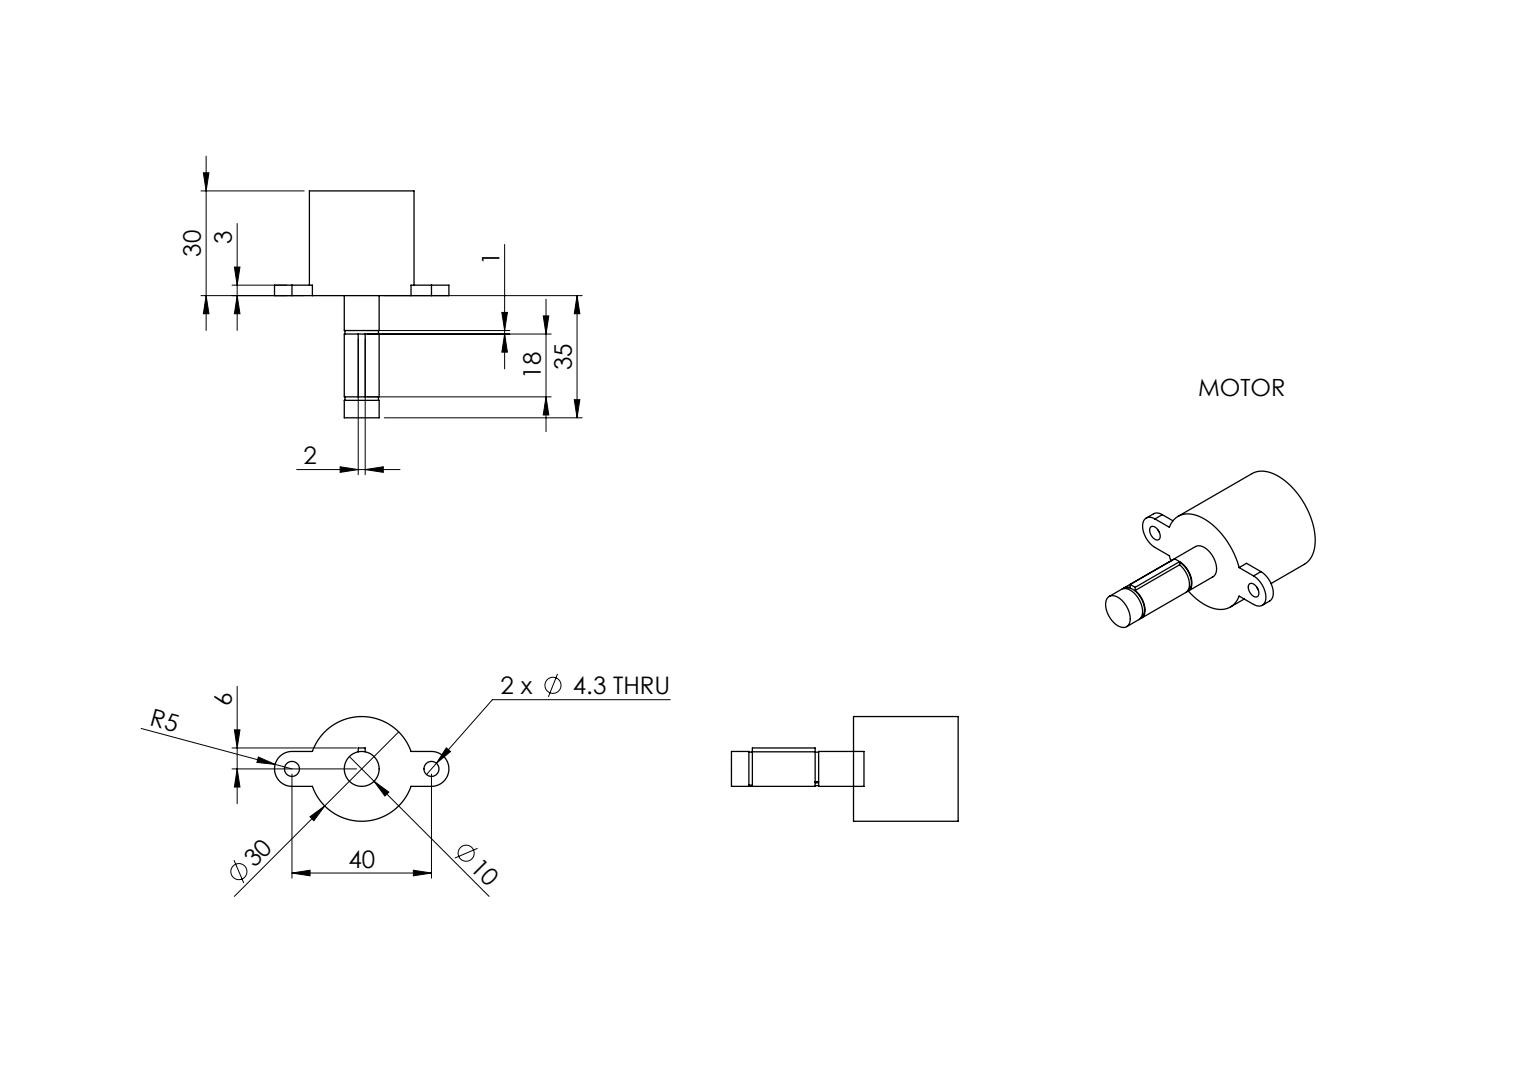
ISO-10303-21;
HEADER;
FILE_DESCRIPTION (('STEP AP214'),
    '1' );
FILE_NAME ('motor.step',
    '2026-10-25T07:12:54',
    ( '' ),
    ( '' ),
    'SwSTEP 2.0',
    'SolidWorks 2026',
    '' );
FILE_SCHEMA (( 'AUTOMOTIVE_DESIGN' ));
ENDSEC;

DATA;
#9=STYLED_ITEM ( 'NONE', ( #1512 ), #12751 ) ;
#21=AXIS2_PLACEMENT_3D ( 'NONE', #13643, #10746, #12742 ) ;
#28=FACE_OUTER_BOUND ( 'NONE', #7057, .T. ) ;
#30=CARTESIAN_POINT ( 'NONE',  ( 22.14999999999999858, -20.00000000000000000, -23.00000000000000000 ) ) ;
#31=ORIENTED_EDGE ( 'NONE', *, *, #5701, .T. ) ;
#100=AXIS2_PLACEMENT_3D ( 'NONE', #7790, #12001, #438 ) ;
#103=EDGE_CURVE ( 'NONE', #12840, #3906, #7426, .T. ) ;
#104=DIRECTION ( 'NONE',  ( -9.710251638871371392E-17, -5.969973981896233748E-17, -1.000000000000000000 ) ) ;
#108=AXIS2_PLACEMENT_3D ( 'NONE', #135, #10772, #2266 ) ;
#110=CARTESIAN_POINT ( 'NONE',  ( 2.385244779468109755E-15, -20.00000000000000000, -9.999999999999994671 ) ) ;
#118=ORIENTED_EDGE ( 'NONE', *, *, #4262, .T. ) ;
#131=ORIENTED_EDGE ( 'NONE', *, *, #11542, .F. ) ;
#135=CARTESIAN_POINT ( 'NONE',  ( 1.267864665261691752E-11, -20.00000000000000000, 9.999999999999998224 ) ) ;
#148=ORIENTED_EDGE ( 'NONE', *, *, #10663, .F. ) ;
#150=ORIENTED_EDGE ( 'NONE', *, *, #2542, .F. ) ;
#159=DIRECTION ( 'NONE',  ( -1.000000000000000000, 0.000000000000000000, 0.000000000000000000 ) ) ;
#171=PLANE ( 'NONE',  #421 ) ;
#179=ORIENTED_EDGE ( 'NONE', *, *, #103, .F. ) ;
#181=ORIENTED_EDGE ( 'NONE', *, *, #4567, .T. ) ;
#190=FACE_OUTER_BOUND ( 'NONE', #6460, .T. ) ;
#202=CARTESIAN_POINT ( 'NONE',  ( -14.99999999999999822, -19.99999999999999645, -23.00000000000000000 ) ) ;
#217=DIRECTION ( 'NONE',  ( -0.000000000000000000, -0.000000000000000000, -1.000000000000000000 ) ) ;
#229=( GEOMETRIC_REPRESENTATION_CONTEXT ( 3 ) GLOBAL_UNCERTAINTY_ASSIGNED_CONTEXT ( ( #8327 ) ) GLOBAL_UNIT_ASSIGNED_CONTEXT ( ( #1931, #1865, #3739 ) ) REPRESENTATION_CONTEXT ( 'NONE', 'WORKASPACE' ) );
#232=ORIENTED_EDGE ( 'NONE', *, *, #13179, .F. ) ;
#250=DIRECTION ( 'NONE',  ( -0.7581610723493046322, -0.6520673188974834833, 1.125475972357111981E-16 ) ) ;
#260=EDGE_CURVE ( 'NONE', #13554, #4523, #9345, .T. ) ;
#263=ORIENTED_EDGE ( 'NONE', *, *, #4115, .F. ) ;
#281=EDGE_CURVE ( 'NONE', #5149, #3301, #7761, .T. ) ;
#283=CYLINDRICAL_SURFACE ( 'NONE', #7915, 5.000000000000000888 ) ;
#294=CARTESIAN_POINT ( 'NONE',  ( 20.00000000000000000, -20.00000000000000000, -23.00000000000000000 ) ) ;
#331=VERTEX_POINT ( 'NONE', #13575 ) ;
#333=LINE ( 'NONE', #7675, #5864 ) ;
#346=ORIENTED_EDGE ( 'NONE', *, *, #2293, .T. ) ;
#347=VERTEX_POINT ( 'NONE', #8345 ) ;
#360=EDGE_CURVE ( 'NONE', #407, #11356, #13500, .T. ) ;
#381=CARTESIAN_POINT ( 'NONE',  ( -3.734041964264191549, -23.01611183630746638, -9.999999999999994671 ) ) ;
#385=CARTESIAN_POINT ( 'NONE',  ( 1.267864665261691752E-11, -20.00000000000000000, 9.999999999999998224 ) ) ;
#405=ORIENTED_EDGE ( 'NONE', *, *, #12351, .T. ) ;
#406=EDGE_LOOP ( 'NONE', ( #1718, #12566, #1882, #5438, #12135, #10903, #5270, #9079, #3095, #9271, #9064, #5318 ) ) ;
#407=VERTEX_POINT ( 'NONE', #11378 ) ;
#421=AXIS2_PLACEMENT_3D ( 'NONE', #8685, #3491, #5379 ) ;
#424=DIRECTION ( 'NONE',  ( 0.6040472319084893016, -0.7969485188038759604, -1.107688701425240097E-17 ) ) ;
#430=AXIS2_PLACEMENT_3D ( 'NONE', #5828, #10990, #3471 ) ;
#435=DIRECTION ( 'NONE',  ( 0.9829867750086872524, 0.1836763462126260182, -1.475957441759982183E-22 ) ) ;
#438=DIRECTION ( 'NONE',  ( -1.000000000000000000, 1.734723475976806848E-16, 0.000000000000000000 ) ) ;
#445=DIRECTION ( 'NONE',  ( 0.000000000000000000, 0.000000000000000000, -1.000000000000000000 ) ) ;
#470=VECTOR ( 'NONE', #11867, 1000.000000000000000 ) ;
#495=CIRCLE ( 'NONE', #6054, 15.00000000000000000 ) ;
#498=DIRECTION ( 'NONE',  ( 1.000000000000000000, 0.000000000000000000, 0.000000000000000000 ) ) ;
#503=EDGE_CURVE ( 'NONE', #347, #12172, #6338, .T. ) ;
#504=VERTEX_POINT ( 'NONE', #30 ) ;
#512=DIRECTION ( 'NONE',  ( -0.000000000000000000, -0.000000000000000000, 1.000000000000000000 ) ) ;
#520=ORIENTED_EDGE ( 'NONE', *, *, #4096, .T. ) ;
#524=CARTESIAN_POINT ( 'NONE',  ( 1.219878473194463187, -24.84890673354692936, 9.000000000000000000 ) ) ;
#538=ORIENTED_EDGE ( 'NONE', *, *, #13172, .T. ) ;
#542=CARTESIAN_POINT ( 'NONE',  ( 20.00000000000000000, -20.00000000000000000, -23.00000000000000000 ) ) ;
#555=CIRCLE ( 'NONE', #9633, 5.000000000000000888 ) ;
#573=DIRECTION ( 'NONE',  ( -0.000000000000000000, -0.000000000000000000, -1.000000000000000000 ) ) ;
#576=LINE ( 'NONE', #13235, #12689 ) ;
#600=DIRECTION ( 'NONE',  ( -0.000000000000000000, -0.000000000000000000, 1.000000000000000000 ) ) ;
#610=CARTESIAN_POINT ( 'NONE',  ( 2.482347295856823136E-15, -20.00000000000000000, -8.999999999999996447 ) ) ;
#623=EDGE_CURVE ( 'NONE', #12722, #6800, #4521, .T. ) ;
#651=VERTEX_POINT ( 'NONE', #1248 ) ;
#653=ORIENTED_EDGE ( 'NONE', *, *, #7184, .F. ) ;
#664=ADVANCED_FACE ( 'NONE', ( #7703 ), #11843, .F. ) ;
#666=VECTOR ( 'NONE', #1055, 1000.000000000000000 ) ;
#683=VECTOR ( 'NONE', #512, 1000.000000000000000 ) ;
#690=VERTEX_POINT ( 'NONE', #9775 ) ;
#692=CIRCLE ( 'NONE', #11545, 2.149999999999999023 ) ;
#705=ORIENTED_EDGE ( 'NONE', *, *, #6210, .F. ) ;
#706=EDGE_CURVE ( 'NONE', #10906, #10425, #3298, .T. ) ;
#711=DIRECTION ( 'NONE',  ( -0.7779254092217071648, -0.6283566325640553840, 0.000000000000000000 ) ) ;
#713=CARTESIAN_POINT ( 'NONE',  ( -4.999999999999998224, -20.00000000000000000, -20.00000000000000000 ) ) ;
#714=DIRECTION ( 'NONE',  ( -0.7779254092217071648, -0.6283566325640553840, 0.000000000000000000 ) ) ;
#728=LINE ( 'NONE', #11257, #8503 ) ;
#735=DIRECTION ( 'NONE',  ( -1.000000000000000000, 0.000000000000000000, 0.000000000000000000 ) ) ;
#739=CIRCLE ( 'NONE', #6941, 5.000000000000000888 ) ;
#742=VECTOR ( 'NONE', #13525, 1000.000000000000000 ) ;
#743=LINE ( 'NONE', #9777, #4835 ) ;
#757=VERTEX_POINT ( 'NONE', #9640 ) ;
#781=CARTESIAN_POINT ( 'NONE',  ( 2.449293598294706513E-15, -20.00000000000000000, -20.00000000000000000 ) ) ;
#784=CARTESIAN_POINT ( 'NONE',  ( 0.8816464618332836567, -24.71833652004169934, 9.999999999999998224 ) ) ;
#790=DIRECTION ( 'NONE',  ( -1.000000000000000000, 0.000000000000000000, 0.000000000000000000 ) ) ;
#800=CARTESIAN_POINT ( 'NONE',  ( 4.688877333453708829, -18.97314589549297281, 9.999999999999998224 ) ) ;
#809=ORIENTED_EDGE ( 'NONE', *, *, #4115, .T. ) ;
#813=CYLINDRICAL_SURFACE ( 'NONE', #10822, 2.149999999999999023 ) ;
#823=ORIENTED_EDGE ( 'NONE', *, *, #3310, .T. ) ;
#824=ORIENTED_EDGE ( 'NONE', *, *, #3992, .T. ) ;
#842=CARTESIAN_POINT ( 'NONE',  ( 14.14213562373095101, -25.00000000000000711, -50.00000000000000000 ) ) ;
#845=ORIENTED_EDGE ( 'NONE', *, *, #3310, .F. ) ;
#849=EDGE_CURVE ( 'NONE', #12479, #12223, #1301, .T. ) ;
#864=EDGE_LOOP ( 'NONE', ( #11730, #7424, #1233, #7744 ) ) ;
#869=CARTESIAN_POINT ( 'NONE',  ( 0.9183817310753817909, -24.91493387504115020, 9.999999999999998224 ) ) ;
#902=DIRECTION ( 'NONE',  ( -1.000000000000000000, 0.000000000000000000, 0.000000000000000000 ) ) ;
#910=EDGE_CURVE ( 'NONE', #11255, #13173, #3889, .T. ) ;
#963=VECTOR ( 'NONE', #11375, 1000.000000000000000 ) ;
#990=ADVANCED_FACE ( 'NONE', ( #9245 ), #7176, .T. ) ;
#995=EDGE_CURVE ( 'NONE', #3770, #10955, #495, .T. ) ;
#1005=DIRECTION ( 'NONE',  ( 0.000000000000000000, 0.000000000000000000, -1.000000000000000000 ) ) ;
#1007=CARTESIAN_POINT ( 'NONE',  ( -20.00000000000000000, -19.99999999999999289, -23.00000000000000000 ) ) ;
#1011=PRODUCT ( 'motor', 'motor', '', ( #7156 ) ) ;
#1012=DIRECTION ( 'NONE',  ( -9.858538378746663627E-23, 5.031452844637890958E-23, -1.000000000000000000 ) ) ;
#1020=CARTESIAN_POINT ( 'NONE',  ( 3.020236159542449172, -23.98474259401938014, -8.999999999999998224 ) ) ;
#1032=EDGE_LOOP ( 'NONE', ( #8046, #6869, #12318, #1285 ) ) ;
#1047=FACE_OUTER_BOUND ( 'NONE', #2834, .T. ) ;
#1048=ORIENTED_EDGE ( 'NONE', *, *, #6072, .F. ) ;
#1055=DIRECTION ( 'NONE',  ( 0.000000000000000000, 0.000000000000000000, 1.000000000000000000 ) ) ;
#1081=ORIENTED_EDGE ( 'NONE', *, *, #7273, .T. ) ;
#1082=ORIENTED_EDGE ( 'NONE', *, *, #503, .T. ) ;
#1084=CARTESIAN_POINT ( 'NONE',  ( 20.00000000000000000, -14.99999999999999289, -20.00000000000000000 ) ) ;
#1088=AXIS2_PLACEMENT_3D ( 'NONE', #1977, #9515, #7322 ) ;
#1102=DIRECTION ( 'NONE',  ( -9.858538378746663627E-23, 5.031452844637890958E-23, -1.000000000000000000 ) ) ;
#1106=DIRECTION ( 'NONE',  ( -1.000000000000000000, 0.000000000000000000, 0.000000000000000000 ) ) ;
#1110=VECTOR ( 'NONE', #8764, 1000.000000000000000 ) ;
#1115=DIRECTION ( 'NONE',  ( 0.000000000000000000, 1.000000000000000000, 0.000000000000000000 ) ) ;
#1139=ORIENTED_EDGE ( 'NONE', *, *, #8132, .T. ) ;
#1170=ORIENTED_EDGE ( 'NONE', *, *, #7701, .F. ) ;
#1175=VECTOR ( 'NONE', #104, 1000.000000000000000 ) ;
#1182=CARTESIAN_POINT ( 'NONE',  ( -17.85000000000000142, -19.99999999999999289, -20.00000000000000000 ) ) ;
#1190=EDGE_LOOP ( 'NONE', ( #2623, #5170, #4957, #13127 ) ) ;
#1199=AXIS2_PLACEMENT_3D ( 'NONE', #9457, #9400, #13594 ) ;
#1203=CARTESIAN_POINT ( 'NONE',  ( 20.00000000000000000, -25.00000000000000711, -23.00000000000000000 ) ) ;
#1204=DIRECTION ( 'NONE',  ( -0.000000000000000000, -0.000000000000000000, -1.000000000000000000 ) ) ;
#1209=EDGE_LOOP ( 'NONE', ( #4886, #9308, #8557, #1048 ) ) ;
#1233=ORIENTED_EDGE ( 'NONE', *, *, #3769, .T. ) ;
#1248=CARTESIAN_POINT ( 'NONE',  ( 1.219878473194463187, -24.84890673354692936, 9.999999999999998224 ) ) ;
#1251=DIRECTION ( 'NONE',  ( -0.2439756946365075896, 0.9697813467099856144, 1.610118993450814692E-22 ) ) ;
#1264=EDGE_LOOP ( 'NONE', ( #3888, #6058, #2553, #520 ) ) ;
#1285=ORIENTED_EDGE ( 'NONE', *, *, #3067, .F. ) ;
#1293=CARTESIAN_POINT ( 'NONE',  ( 5.000000000000003553, -20.00000000000000000, -20.00000000000000000 ) ) ;
#1301=CIRCLE ( 'NONE', #13223, 5.000000000000007994 ) ;
#1306=CARTESIAN_POINT ( 'NONE',  ( 1.267864665261691752E-11, -20.00000000000000000, 9.999999999999998224 ) ) ;
#1322=DIRECTION ( 'NONE',  ( 0.000000000000000000, 0.000000000000000000, -1.000000000000000000 ) ) ;
#1324=CARTESIAN_POINT ( 'NONE',  ( -17.85000000000000142, -19.99999999999999289, -23.00000000000000000 ) ) ;
#1334=ORIENTED_EDGE ( 'NONE', *, *, #4336, .T. ) ;
#1357=CIRCLE ( 'NONE', #4686, 2.149999999999999023 ) ;
#1360=DIRECTION ( 'NONE',  ( -0.7779254092217071648, -0.6283566325640553840, 0.000000000000000000 ) ) ;
#1385=DIRECTION ( 'NONE',  ( 1.000000000000000000, -1.734723475976807341E-16, -0.000000000000000000 ) ) ;
#1388=CARTESIAN_POINT ( 'NONE',  ( 2.899426713160750069, -23.82535289025860337, -9.999999999999994671 ) ) ;
#1395=PLANE ( 'NONE',  #11068 ) ;
#1408=AXIS2_PLACEMENT_3D ( 'NONE', #6301, #1005, #7116 ) ;
#1416=DIRECTION ( 'NONE',  ( 0.6040472319084893016, -0.7969485188038759604, -1.107688701425240251E-17 ) ) ;
#1421=VERTEX_POINT ( 'NONE', #12715 ) ;
#1434=ORIENTED_EDGE ( 'NONE', *, *, #9580, .T. ) ;
#1467=PLANE ( 'NONE',  #5074 ) ;
#1473=ORIENTED_EDGE ( 'NONE', *, *, #11540, .F. ) ;
#1489=VERTEX_POINT ( 'NONE', #2987 ) ;
#1492=FACE_OUTER_BOUND ( 'NONE', #8858, .T. ) ;
#1499=LINE ( 'NONE', #13053, #9995 ) ;
#1512=PRESENTATION_STYLE_ASSIGNMENT (( #6791 ) ) ;
#1546=CARTESIAN_POINT ( 'NONE',  ( -3.734041964264191549, -23.01611183630746638, -8.999999999999996447 ) ) ;
#1555=VECTOR ( 'NONE', #6821, 999.9999999999998863 ) ;
#1574=EDGE_LOOP ( 'NONE', ( #3279, #705, #2695, #5481, #5837, #7241, #9903, #9024 ) ) ;
#1611=EDGE_CURVE ( 'NONE', #13245, #504, #728, .T. ) ;
#1620=AXIS2_PLACEMENT_3D ( 'NONE', #4593, #5570, #8747 ) ;
#1628=AXIS2_PLACEMENT_3D ( 'NONE', #13208, #1322, #6741 ) ;
#1646=ORIENTED_EDGE ( 'NONE', *, *, #12351, .F. ) ;
#1669=CIRCLE ( 'NONE', #5891, 4.799999999999999822 ) ;
#1678=CARTESIAN_POINT ( 'NONE',  ( 20.00000000000000000, -25.00000000000000711, -23.00000000000000000 ) ) ;
#1681=ORIENTED_EDGE ( 'NONE', *, *, #5603, .T. ) ;
#1693=EDGE_CURVE ( 'NONE', #4523, #12971, #6022, .T. ) ;
#1697=EDGE_CURVE ( 'NONE', #5890, #11555, #12498, .T. ) ;
#1704=CARTESIAN_POINT ( 'NONE',  ( 17.85000000000000142, -20.00000000000000000, -23.00000000000000000 ) ) ;
#1708=EDGE_CURVE ( 'NONE', #9272, #8675, #5122, .T. ) ;
#1716=EDGE_LOOP ( 'NONE', ( #232, #7425, #4993, #9885, #7605, #12254, #2606, #5059 ) ) ;
#1718=ORIENTED_EDGE ( 'NONE', *, *, #1708, .F. ) ;
#1719=DIRECTION ( 'NONE',  ( -1.000000000000000000, 0.000000000000000000, 0.000000000000000000 ) ) ;
#1720=LINE ( 'NONE', #9068, #8575 ) ;
#1728=ADVANCED_FACE ( 'NONE', ( #12363 ), #6303, .T. ) ;
#1730=DIRECTION ( 'NONE',  ( -0.2439756946365075896, 0.9697813467099857254, 1.610118993450814692E-22 ) ) ;
#1738=EDGE_LOOP ( 'NONE', ( #9969, #12992 ) ) ;
#1741=SHAPE_DEFINITION_REPRESENTATION ( #12618, #11036 ) ;
#1745=CARTESIAN_POINT ( 'NONE',  ( 2.482347295856823136E-15, -20.00000000000000000, -8.999999999999996447 ) ) ;
#1787=VERTEX_POINT ( 'NONE', #3373 ) ;
#1790=AXIS2_PLACEMENT_3D ( 'NONE', #10437, #10100, #13603 ) ;
#1808=EDGE_LOOP ( 'NONE', ( #1646, #10556, #3839, #4401 ) ) ;
#1819=LINE ( 'NONE', #10329, #2792 ) ;
#1825=AXIS2_PLACEMENT_3D ( 'NONE', #8022, #3667, #7954 ) ;
#1827=EDGE_LOOP ( 'NONE', ( #3789, #7685, #4973, #11985 ) ) ;
#1828=DIRECTION ( 'NONE',  ( 0.000000000000000000, 0.000000000000000000, 1.000000000000000000 ) ) ;
#1840=ORIENTED_EDGE ( 'NONE', *, *, #2185, .F. ) ;
#1844=DIRECTION ( 'NONE',  ( -0.000000000000000000, -0.000000000000000000, -1.000000000000000000 ) ) ;
#1855=CIRCLE ( 'NONE', #5189, 4.800000000000000711 ) ;
#1865=( NAMED_UNIT ( * ) PLANE_ANGLE_UNIT ( ) SI_UNIT ( $, .RADIAN. ) );
#1868=FACE_OUTER_BOUND ( 'NONE', #1808, .T. ) ;
#1880=VECTOR ( 'NONE', #6757, 1000.000000000000000 ) ;
#1882=ORIENTED_EDGE ( 'NONE', *, *, #8132, .F. ) ;
#1885=CARTESIAN_POINT ( 'NONE',  ( 2.449293598294706513E-15, -20.00000000000000000, 15.00000000000000355 ) ) ;
#1896=DIRECTION ( 'NONE',  ( -1.000000000000000000, 0.000000000000000000, 0.000000000000000000 ) ) ;
#1897=ORIENTED_EDGE ( 'NONE', *, *, #7519, .T. ) ;
#1899=DIRECTION ( 'NONE',  ( 1.000000000000000000, 0.000000000000000000, 0.000000000000000000 ) ) ;
#1916=DIRECTION ( 'NONE',  ( -1.000000000000000000, 0.000000000000000000, 0.000000000000000000 ) ) ;
#1930=VECTOR ( 'NONE', #7556, 1000.000000000000000 ) ;
#1931=( LENGTH_UNIT ( ) NAMED_UNIT ( * ) SI_UNIT ( .MILLI., .METRE. ) );
#1937=ADVANCED_FACE ( 'NONE', ( #6562, #10762, #4278, #11609 ), #6367, .F. ) ;
#1941=ORIENTED_EDGE ( 'NONE', *, *, #3233, .F. ) ;
#1950=DIRECTION ( 'NONE',  ( 0.000000000000000000, 0.000000000000000000, -1.000000000000000000 ) ) ;
#1972=AXIS2_PLACEMENT_3D ( 'NONE', #3079, #6284, #1896 ) ;
#1977=CARTESIAN_POINT ( 'NONE',  ( 2.449293598294706513E-15, -20.00000000000000000, 15.00000000000000355 ) ) ;
#1987=FACE_OUTER_BOUND ( 'NONE', #1190, .T. ) ;
#1988=AXIS2_PLACEMENT_3D ( 'NONE', #7337, #1012, #3309 ) ;
#1989=ORIENTED_EDGE ( 'NONE', *, *, #11540, .T. ) ;
#2013=EDGE_CURVE ( 'NONE', #5545, #4887, #2463, .T. ) ;
#2015=ORIENTED_EDGE ( 'NONE', *, *, #2346, .F. ) ;
#2034=CYLINDRICAL_SURFACE ( 'NONE', #5843, 4.800000000000000711 ) ;
#2042=CYLINDRICAL_SURFACE ( 'NONE', #21, 4.799999999999999822 ) ;
#2070=CARTESIAN_POINT ( 'NONE',  ( -0.9999999999999995559, -15.10102051443364246, 15.00000000000000355 ) ) ;
#2088=AXIS2_PLACEMENT_3D ( 'NONE', #10550, #3091, #790 ) ;
#2098=CARTESIAN_POINT ( 'NONE',  ( 1.267864665261691752E-11, -20.00000000000000000, 9.999999999999998224 ) ) ;
#2109=EDGE_CURVE ( 'NONE', #10425, #12479, #6894, .T. ) ;
#2134=CARTESIAN_POINT ( 'NONE',  ( 2.899426713160750069, -23.82535289025860337, -8.999999999999996447 ) ) ;
#2169=FACE_OUTER_BOUND ( 'NONE', #7043, .T. ) ;
#2181=EDGE_LOOP ( 'NONE', ( #3330, #12040, #2890, #2015 ) ) ;
#2185=EDGE_CURVE ( 'NONE', #1787, #12223, #12747, .T. ) ;
#2188=FACE_OUTER_BOUND ( 'NONE', #13311, .T. ) ;
#2214=AXIS2_PLACEMENT_3D ( 'NONE', #10842, #9748, #7676 ) ;
#2225=CARTESIAN_POINT ( 'NONE',  ( 17.85000000000000142, -20.00000000000000000, -23.00000000000000000 ) ) ;
#2233=CARTESIAN_POINT ( 'NONE',  ( 14.14213562373095101, -25.00000000000000711, -23.00000000000000000 ) ) ;
#2234=AXIS2_PLACEMENT_3D ( 'NONE', #7626, #8735, #6727 ) ;
#2242=DIRECTION ( 'NONE',  ( -1.000000000000000000, 0.000000000000000000, 0.000000000000000000 ) ) ;
#2266=DIRECTION ( 'NONE',  ( -0.9768494444668812671, -0.2139279384389642935, 0.000000000000000000 ) ) ;
#2267=CARTESIAN_POINT ( 'NONE',  ( -1.000000000000000000, -14.00000000000000000, 8.999999999999998224 ) ) ;
#2282=ADVANCED_FACE ( 'NONE', ( #10880 ), #1395, .F. ) ;
#2284=CIRCLE ( 'NONE', #10239, 5.000000000000007994 ) ;
#2290=EDGE_CURVE ( 'NONE', #6976, #8572, #4455, .T. ) ;
#2293=EDGE_CURVE ( 'NONE', #11760, #5079, #4909, .T. ) ;
#2298=VECTOR ( 'NONE', #9222, 1000.000000000000000 ) ;
#2300=ADVANCED_FACE ( 'NONE', ( #11997 ), #12882, .T. ) ;
#2305=DIRECTION ( 'NONE',  ( -0.9697813467099857254, -0.2439756946365076173, 1.379242460255691792E-22 ) ) ;
#2346=EDGE_CURVE ( 'NONE', #4780, #6905, #13357, .T. ) ;
#2347=ORIENTED_EDGE ( 'NONE', *, *, #10264, .F. ) ;
#2349=ORIENTED_EDGE ( 'NONE', *, *, #7292, .F. ) ;
#2392=AXIS2_PLACEMENT_3D ( 'NONE', #10166, #11198, #1719 ) ;
#2400=ORIENTED_EDGE ( 'NONE', *, *, #13346, .F. ) ;
#2420=VECTOR ( 'NONE', #2954, 1000.000000000000000 ) ;
#2427=EDGE_CURVE ( 'NONE', #5888, #11823, #1669, .T. ) ;
#2432=AXIS2_PLACEMENT_3D ( 'NONE', #6382, #10446, #3255 ) ;
#2437=DIRECTION ( 'NONE',  ( -0.000000000000000000, -0.000000000000000000, -1.000000000000000000 ) ) ;
#2463=CIRCLE ( 'NONE', #3137, 2.149999999999999023 ) ;
#2500=DIRECTION ( 'NONE',  ( -1.734723475976807341E-16, -1.000000000000000000, 0.000000000000000000 ) ) ;
#2521=AXIS2_PLACEMENT_3D ( 'NONE', #1007, #9459, #8431 ) ;
#2526=CARTESIAN_POINT ( 'NONE',  ( 5.000000000000003553, -20.00000000000000000, -9.999999999999994671 ) ) ;
#2529=EDGE_CURVE ( 'NONE', #4887, #5545, #12500, .T. ) ;
#2542=EDGE_CURVE ( 'NONE', #9150, #5892, #555, .T. ) ;
#2543=DIRECTION ( 'NONE',  ( 0.000000000000000000, 0.000000000000000000, -1.000000000000000000 ) ) ;
#2553=ORIENTED_EDGE ( 'NONE', *, *, #10454, .T. ) ;
#2556=ORIENTED_EDGE ( 'NONE', *, *, #4759, .F. ) ;
#2562=SURFACE_SIDE_STYLE ('',( #8865 ) ) ;
#2569=CARTESIAN_POINT ( 'NONE',  ( 20.00000000000000000, -14.99999999999999289, -23.00000000000000000 ) ) ;
#2574=CARTESIAN_POINT ( 'NONE',  ( 20.00000000000000000, -20.00000000000000000, -20.00000000000000000 ) ) ;
#2578=CARTESIAN_POINT ( 'NONE',  ( 1.267864665251833278E-11, -20.00000000000000000, 9.000000000000000000 ) ) ;
#2583=DIRECTION ( 'NONE',  ( -0.7779254092217071648, -0.6283566325640553840, 0.000000000000000000 ) ) ;
#2591=DIRECTION ( 'NONE',  ( -1.000000000000000000, 0.000000000000000000, 0.000000000000000000 ) ) ;
#2603=AXIS2_PLACEMENT_3D ( 'NONE', #8934, #600, #13263 ) ;
#2606=ORIENTED_EDGE ( 'NONE', *, *, #995, .T. ) ;
#2614=CYLINDRICAL_SURFACE ( 'NONE', #6233, 15.00000000000000000 ) ;
#2622=AXIS2_PLACEMENT_3D ( 'NONE', #11016, #12266, #3968 ) ;
#2623=ORIENTED_EDGE ( 'NONE', *, *, #1697, .T. ) ;
#2624=ORIENTED_EDGE ( 'NONE', *, *, #6395, .T. ) ;
#2659=ORIENTED_EDGE ( 'NONE', *, *, #2719, .T. ) ;
#2677=VERTEX_POINT ( 'NONE', #13569 ) ;
#2680=ORIENTED_EDGE ( 'NONE', *, *, #4096, .F. ) ;
#2695=ORIENTED_EDGE ( 'NONE', *, *, #7552, .T. ) ;
#2697=ORIENTED_EDGE ( 'NONE', *, *, #8399, .T. ) ;
#2698=DIRECTION ( 'NONE',  ( -0.000000000000000000, -0.000000000000000000, 1.000000000000000000 ) ) ;
#2711=VERTEX_POINT ( 'NONE', #9229 ) ;
#2719=EDGE_CURVE ( 'NONE', #11823, #11760, #1819, .T. ) ;
#2746=AXIS2_PLACEMENT_3D ( 'NONE', #11584, #1115, #13429 ) ;
#2755=ORIENTED_EDGE ( 'NONE', *, *, #12525, .T. ) ;
#2771=VERTEX_POINT ( 'NONE', #1182 ) ;
#2789=VERTEX_POINT ( 'NONE', #5559 ) ;
#2792=VECTOR ( 'NONE', #6065, 1000.000000000000114 ) ;
#2813=CARTESIAN_POINT ( 'NONE',  ( 2.449293598294706513E-15, -20.00000000000000000, -23.00000000000000000 ) ) ;
#2834=EDGE_LOOP ( 'NONE', ( #10782, #13044, #1897, #7724 ) ) ;
#2840=FACE_OUTER_BOUND ( 'NONE', #9132, .T. ) ;
#2850=AXIS2_PLACEMENT_3D ( 'NONE', #8753, #11789, #9651 ) ;
#2853=DIRECTION ( 'NONE',  ( 0.000000000000000000, 0.000000000000000000, -1.000000000000000000 ) ) ;
#2870=DIRECTION ( 'NONE',  ( -0.000000000000000000, -0.000000000000000000, 1.000000000000000000 ) ) ;
#2890=ORIENTED_EDGE ( 'NONE', *, *, #10531, .T. ) ;
#2891=CARTESIAN_POINT ( 'NONE',  ( 20.00000000000000000, -14.99999999999999289, -23.00000000000000000 ) ) ;
#2900=DIRECTION ( 'NONE',  ( -0.000000000000000000, -0.000000000000000000, 1.000000000000000000 ) ) ;
#2908=ORIENTED_EDGE ( 'NONE', *, *, #3602, .T. ) ;
#2912=FACE_BOUND ( 'NONE', #1738, .T. ) ;
#2936=CARTESIAN_POINT ( 'NONE',  ( -22.14999999999999858, -19.99999999999999289, -23.00000000000000000 ) ) ;
#2943=CIRCLE ( 'NONE', #1825, 5.000000000000000888 ) ;
#2949=DIRECTION ( 'NONE',  ( -1.000000000000000000, -4.082155997157843695E-16, 0.000000000000000000 ) ) ;
#2950=CLOSED_SHELL ( 'NONE', ( #6174, #8344, #9664, #6098, #2981, #7491, #8600, #10497, #7205, #10910, #2300, #9930, #10273, #9322, #11759, #1937, #1728, #8370, #10770, #3896, #7071, #10494, #5349, #10066, #7769, #664, #7458, #4338, #6200, #6808, #7135, #9712, #2282, #990, #13011, #6166, #10063, #4236, #5363, #5115 ) ) ;
#2954=DIRECTION ( 'NONE',  ( -9.858538378746663627E-23, 5.031452844637890958E-23, -1.000000000000000000 ) ) ;
#2974=VECTOR ( 'NONE', #8259, 1000.000000000000000 ) ;
#2981=ADVANCED_FACE ( 'NONE', ( #4725 ), #5835, .T. ) ;
#2987=CARTESIAN_POINT ( 'NONE',  ( -20.00000000000000000, -25.00000000000000000, -20.00000000000000000 ) ) ;
#3018=PLANE ( 'NONE',  #6000 ) ;
#3026=ORIENTED_EDGE ( 'NONE', *, *, #9719, .T. ) ;
#3031=CARTESIAN_POINT ( 'NONE',  ( 2.449293598294706513E-15, -20.00000000000000000, -20.00000000000000000 ) ) ;
#3054=VECTOR ( 'NONE', #7812, 1000.000000000000000 ) ;
#3062=CARTESIAN_POINT ( 'NONE',  ( -4.999999999999998224, -20.00000000000000000, 15.00000000000000355 ) ) ;
#3067=EDGE_CURVE ( 'NONE', #690, #1489, #13074, .T. ) ;
#3077=ORIENTED_EDGE ( 'NONE', *, *, #13406, .T. ) ;
#3079=CARTESIAN_POINT ( 'NONE',  ( 2.449293598294706513E-15, -20.00000000000000000, 9.000000000000000000 ) ) ;
#3082=ORIENTED_EDGE ( 'NONE', *, *, #5188, .F. ) ;
#3083=CARTESIAN_POINT ( 'NONE',  ( 2.449293598294706513E-15, -20.00000000000000000, -23.00000000000000000 ) ) ;
#3085=DIRECTION ( 'NONE',  ( -9.858538378746663627E-23, 5.031452844637890958E-23, -1.000000000000000000 ) ) ;
#3091=DIRECTION ( 'NONE',  ( -9.710251638871371392E-17, -5.969973981896233748E-17, -1.000000000000000000 ) ) ;
#3095=ORIENTED_EDGE ( 'NONE', *, *, #503, .F. ) ;
#3137=AXIS2_PLACEMENT_3D ( 'NONE', #6761, #573, #9994 ) ;
#3147=VERTEX_POINT ( 'NONE', #10178 ) ;
#3170=EDGE_CURVE ( 'NONE', #10837, #331, #11981, .T. ) ;
#3179=AXIS2_PLACEMENT_3D ( 'NONE', #11237, #4962, #711 ) ;
#3218=ORIENTED_EDGE ( 'NONE', *, *, #13008, .F. ) ;
#3233=EDGE_CURVE ( 'NONE', #7327, #9150, #8320, .T. ) ;
#3234=ORIENTED_EDGE ( 'NONE', *, *, #623, .F. ) ;
#3239=CARTESIAN_POINT ( 'NONE',  ( 1.171083334267915221, -24.65495046420793201, 9.000000000000000000 ) ) ;
#3246=EDGE_CURVE ( 'NONE', #331, #10837, #4038, .T. ) ;
#3255=DIRECTION ( 'NONE',  ( -1.000000000000000000, 0.000000000000000000, 0.000000000000000000 ) ) ;
#3265=EDGE_LOOP ( 'NONE', ( #8290, #11231, #5908, #5824 ) ) ;
#3279=ORIENTED_EDGE ( 'NONE', *, *, #11433, .F. ) ;
#3280=CARTESIAN_POINT ( 'NONE',  ( 1.000000000000002442, -20.00000000000000000, 8.999999999999998224 ) ) ;
#3291=DIRECTION ( 'NONE',  ( -9.710251638871371392E-17, -5.969973981896234981E-17, -1.000000000000000000 ) ) ;
#3298=CIRCLE ( 'NONE', #12126, 5.000000000000007994 ) ;
#3300=VERTEX_POINT ( 'NONE', #7481 ) ;
#3301=VERTEX_POINT ( 'NONE', #8449 ) ;
#3309=DIRECTION ( 'NONE',  ( -1.000000000000000000, 0.000000000000000000, 0.000000000000000000 ) ) ;
#3310=EDGE_CURVE ( 'NONE', #757, #1421, #12783, .T. ) ;
#3330=ORIENTED_EDGE ( 'NONE', *, *, #10658, .F. ) ;
#3331=EDGE_LOOP ( 'NONE', ( #9117, #10285, #6836, #2680, #3234, #8758, #8426, #4013, #8427 ) ) ;
#3342=CARTESIAN_POINT ( 'NONE',  ( 3.734041964264196878, -16.98388816369253362, -8.999999999999996447 ) ) ;
#3352=CARTESIAN_POINT ( 'NONE',  ( 1.171083334267915221, -24.65495046420793201, 9.999999999999998224 ) ) ;
#3353=AXIS2_PLACEMENT_3D ( 'NONE', #10621, #6487, #3428 ) ;
#3373=CARTESIAN_POINT ( 'NONE',  ( 20.00000000000000000, -25.00000000000000711, -23.00000000000000000 ) ) ;
#3380=AXIS2_PLACEMENT_3D ( 'NONE', #1306, #6461, #10724 ) ;
#3386=DIRECTION ( 'NONE',  ( -0.000000000000000000, -0.000000000000000000, -1.000000000000000000 ) ) ;
#3408=CIRCLE ( 'NONE', #7837, 5.000000000000007994 ) ;
#3428=DIRECTION ( 'NONE',  ( -1.000000000000000000, 0.000000000000000000, 0.000000000000000000 ) ) ;
#3431=DIRECTION ( 'NONE',  ( -1.000000000000000000, 0.000000000000000000, 0.000000000000000000 ) ) ;
#3458=CARTESIAN_POINT ( 'NONE',  ( -1.000000000000000000, -14.00000000000000000, 8.999999999999998224 ) ) ;
#3462=CARTESIAN_POINT ( 'NONE',  ( 3.129923130707922496, -23.63917314727666152, -8.999999999999996447 ) ) ;
#3470=LINE ( 'NONE', #7762, #1930 ) ;
#3471=DIRECTION ( 'NONE',  ( 1.000000000000000000, 0.000000000000000000, 0.000000000000000000 ) ) ;
#3479=EDGE_CURVE ( 'NONE', #10164, #7327, #2943, .T. ) ;
#3491=DIRECTION ( 'NONE',  ( -1.545477659731174253E-22, 3.805888647522192075E-23, -1.000000000000000000 ) ) ;
#3500=ORIENTED_EDGE ( 'NONE', *, *, #13206, .F. ) ;
#3502=CIRCLE ( 'NONE', #11460, 5.000000000000000888 ) ;
#3517=EDGE_LOOP ( 'NONE', ( #5686, #6143 ) ) ;
#3528=CIRCLE ( 'NONE', #9706, 4.799999999999999822 ) ;
#3544=APPLICATION_CONTEXT ( 'automotive_design' ) ;
#3556=VECTOR ( 'NONE', #9975, 1000.000000000000000 ) ;
#3560=EDGE_CURVE ( 'NONE', #9611, #13146, #1499, .T. ) ;
#3588=CARTESIAN_POINT ( 'NONE',  ( 1.000000000000002442, -20.00000000000000000, 8.999999999999998224 ) ) ;
#3602=EDGE_CURVE ( 'NONE', #6107, #9574, #6492, .T. ) ;
#3611=DIRECTION ( 'NONE',  ( 1.000000000000000000, -1.734723475976807341E-16, -0.000000000000000000 ) ) ;
#3615=DIRECTION ( 'NONE',  ( 9.710251638871371392E-17, 5.969973981896233748E-17, 1.000000000000000000 ) ) ;
#3644=CARTESIAN_POINT ( 'NONE',  ( -20.00000000000000000, -19.99999999999999289, -20.00000000000000000 ) ) ;
#3656=EDGE_LOOP ( 'NONE', ( #12645, #6036, #4122, #11341 ) ) ;
#3667=DIRECTION ( 'NONE',  ( -9.710251638871371392E-17, -5.969973981896233748E-17, -1.000000000000000000 ) ) ;
#3688=CARTESIAN_POINT ( 'NONE',  ( -14.14213562373094213, -14.99999999999998757, -23.00000000000000000 ) ) ;
#3702=CARTESIAN_POINT ( 'NONE',  ( 15.00000000000000178, -20.00000000000000000, -23.00000000000000000 ) ) ;
#3705=CARTESIAN_POINT ( 'NONE',  ( 2.449293598294706513E-15, -20.00000000000000000, 15.00000000000000355 ) ) ;
#3718=CARTESIAN_POINT ( 'NONE',  ( -14.14213562373094213, -14.99999999999998757, -50.00000000000000000 ) ) ;
#3739=( NAMED_UNIT ( * ) SI_UNIT ( $, .STERADIAN. ) SOLID_ANGLE_UNIT ( ) );
#3742=EDGE_CURVE ( 'NONE', #12223, #407, #10368, .T. ) ;
#3755=EDGE_LOOP ( 'NONE', ( #3082, #10073, #824, #6572, #8824, #1139, #9357, #10974, #1989, #6075, #5455, #8743, #1941, #5042, #12056, #6328, #5172, #1082, #5616, #9808 ) ) ;
#3757=DIRECTION ( 'NONE',  ( -1.000000000000000000, 0.000000000000000000, 0.000000000000000000 ) ) ;
#3769=EDGE_CURVE ( 'NONE', #1421, #2711, #5056, .T. ) ;
#3770=VERTEX_POINT ( 'NONE', #4081 ) ;
#3781=DIRECTION ( 'NONE',  ( 1.000000000000000000, 0.000000000000000000, 0.000000000000000000 ) ) ;
#3789=ORIENTED_EDGE ( 'NONE', *, *, #6654, .F. ) ;
#3792=VECTOR ( 'NONE', #11808, 999.9999999999998863 ) ;
#3817=EDGE_CURVE ( 'NONE', #2789, #757, #8823, .T. ) ;
#3819=AXIS2_PLACEMENT_3D ( 'NONE', #8180, #5218, #3884 ) ;
#3834=CARTESIAN_POINT ( 'NONE',  ( -20.00000000000000000, -19.99999999999999289, -23.00000000000000000 ) ) ;
#3837=DIRECTION ( 'NONE',  ( 0.000000000000000000, 0.000000000000000000, -1.000000000000000000 ) ) ;
#3839=ORIENTED_EDGE ( 'NONE', *, *, #10737, .T. ) ;
#3844=CARTESIAN_POINT ( 'NONE',  ( -3.734041964264191549, -23.01611183630746638, -8.999999999999996447 ) ) ;
#3860=ORIENTED_EDGE ( 'NONE', *, *, #11926, .T. ) ;
#3884=DIRECTION ( 'NONE',  ( 1.000000000000000000, 0.000000000000000000, 0.000000000000000000 ) ) ;
#3888=ORIENTED_EDGE ( 'NONE', *, *, #2109, .F. ) ;
#3889=LINE ( 'NONE', #7077, #9049 ) ;
#3890=ORIENTED_EDGE ( 'NONE', *, *, #11945, .T. ) ;
#3893=DIRECTION ( 'NONE',  ( 0.000000000000000000, 0.000000000000000000, -1.000000000000000000 ) ) ;
#3896=ADVANCED_FACE ( 'NONE', ( #4605 ), #11925, .F. ) ;
#3901=CYLINDRICAL_SURFACE ( 'NONE', #5733, 2.149999999999999023 ) ;
#3906=VERTEX_POINT ( 'NONE', #12819 ) ;
#3913=( NAMED_UNIT ( * ) PLANE_ANGLE_UNIT ( ) SI_UNIT ( $, .RADIAN. ) );
#3927=DIRECTION ( 'NONE',  ( -1.000000000000000000, 0.000000000000000000, 0.000000000000000000 ) ) ;
#3944=CARTESIAN_POINT ( 'NONE',  ( 2.449293598294706513E-15, -20.00000000000000000, -8.999999999999998224 ) ) ;
#3954=CIRCLE ( 'NONE', #12776, 15.00000000000000000 ) ;
#3956=ORIENTED_EDGE ( 'NONE', *, *, #706, .T. ) ;
#3957=ORIENTED_EDGE ( 'NONE', *, *, #5425, .F. ) ;
#3968=DIRECTION ( 'NONE',  ( -1.000000000000000000, 0.000000000000000000, -0.000000000000000000 ) ) ;
#3980=CARTESIAN_POINT ( 'NONE',  ( -0.9999999999999976685, -20.00000000000000000, 8.999999999999998224 ) ) ;
#3992=EDGE_CURVE ( 'NONE', #10837, #6107, #10267, .T. ) ;
#4009=DIRECTION ( 'NONE',  ( -9.710251638871371392E-17, -5.969973981896233748E-17, -1.000000000000000000 ) ) ;
#4013=ORIENTED_EDGE ( 'NONE', *, *, #7273, .F. ) ;
#4026=AXIS2_PLACEMENT_3D ( 'NONE', #11640, #8598, #159 ) ;
#4038=CIRCLE ( 'NONE', #3819, 5.000000000000000888 ) ;
#4069=ORIENTED_EDGE ( 'NONE', *, *, #1693, .T. ) ;
#4079=LINE ( 'NONE', #4933, #10199 ) ;
#4081=CARTESIAN_POINT ( 'NONE',  ( 14.14213562373094923, -14.99999999999999112, -23.00000000000000000 ) ) ;
#4096=EDGE_CURVE ( 'NONE', #6800, #12479, #3408, .T. ) ;
#4115=EDGE_CURVE ( 'NONE', #1787, #11356, #5856, .T. ) ;
#4119=EDGE_LOOP ( 'NONE', ( #2349, #3077, #4694, #5133 ) ) ;
#4122=ORIENTED_EDGE ( 'NONE', *, *, #2013, .T. ) ;
#4128=DIRECTION ( 'NONE',  ( 4.082155997157843695E-16, -1.000000000000000000, 0.000000000000000000 ) ) ;
#4129=( LENGTH_UNIT ( ) NAMED_UNIT ( * ) SI_UNIT ( .MILLI., .METRE. ) );
#4163=EDGE_CURVE ( 'NONE', #11255, #5890, #13090, .T. ) ;
#4191=CARTESIAN_POINT ( 'NONE',  ( 3.020236159542449172, -23.98474259401938014, -9.999999999999994671 ) ) ;
#4208=PLANE ( 'NONE',  #4663 ) ;
#4214=VECTOR ( 'NONE', #3611, 1000.000000000000000 ) ;
#4219=EDGE_CURVE ( 'NONE', #4643, #12840, #4296, .T. ) ;
#4236=ADVANCED_FACE ( 'NONE', ( #1047 ), #2034, .T. ) ;
#4246=LINE ( 'NONE', #8464, #5347 ) ;
#4260=CARTESIAN_POINT ( 'NONE',  ( 2.899426713160750069, -23.82535289025860337, -8.999999999999996447 ) ) ;
#4262=EDGE_CURVE ( 'NONE', #9574, #651, #739, .T. ) ;
#4277=DIRECTION ( 'NONE',  ( 0.000000000000000000, 0.000000000000000000, -1.000000000000000000 ) ) ;
#4278=FACE_BOUND ( 'NONE', #9027, .T. ) ;
#4285=AXIS2_PLACEMENT_3D ( 'NONE', #3352, #2305, #1251 ) ;
#4286=ORIENTED_EDGE ( 'NONE', *, *, #4219, .T. ) ;
#4296=CIRCLE ( 'NONE', #12677, 4.800000000000000711 ) ;
#4321=ORIENTED_EDGE ( 'NONE', *, *, #3067, .T. ) ;
#4325=LINE ( 'NONE', #10615, #11944 ) ;
#4336=EDGE_CURVE ( 'NONE', #13537, #4887, #6209, .T. ) ;
#4338=ADVANCED_FACE ( 'NONE', ( #28 ), #7375, .T. ) ;
#4353=ORIENTED_EDGE ( 'NONE', *, *, #12603, .T. ) ;
#4385=FACE_OUTER_BOUND ( 'NONE', #6922, .T. ) ;
#4392=CARTESIAN_POINT ( 'NONE',  ( -4.999999999999998224, -20.00000000000000000, 9.999999999999998224 ) ) ;
#4401=ORIENTED_EDGE ( 'NONE', *, *, #5192, .F. ) ;
#4423=CARTESIAN_POINT ( 'NONE',  ( -4.688877333428352223, -21.02685410450703074, 9.000000000000000000 ) ) ;
#4431=ORIENTED_EDGE ( 'NONE', *, *, #7807, .F. ) ;
#4436=DIRECTION ( 'NONE',  ( -1.000000000000000000, 0.000000000000000000, 0.000000000000000000 ) ) ;
#4449=DIRECTION ( 'NONE',  ( 0.000000000000000000, 0.000000000000000000, -1.000000000000000000 ) ) ;
#4450=EDGE_LOOP ( 'NONE', ( #12237, #8510, #6723, #653 ) ) ;
#4454=CARTESIAN_POINT ( 'NONE',  ( 4.688877333453707941, -18.97314589549297281, 9.000000000000000000 ) ) ;
#4455=CIRCLE ( 'NONE', #7548, 4.799999999999999822 ) ;
#4478=AXIS2_PLACEMENT_3D ( 'NONE', #10451, #11281, #8251 ) ;
#4502=EDGE_LOOP ( 'NONE', ( #13380, #7746, #3956, #11568, #809, #6852 ) ) ;
#4512=VECTOR ( 'NONE', #6814, 1000.000000000000000 ) ;
#4515=DIRECTION ( 'NONE',  ( -0.000000000000000000, -0.000000000000000000, -1.000000000000000000 ) ) ;
#4521=LINE ( 'NONE', #10870, #8597 ) ;
#4523=VERTEX_POINT ( 'NONE', #12283 ) ;
#4541=ORIENTED_EDGE ( 'NONE', *, *, #13352, .F. ) ;
#4567=EDGE_CURVE ( 'NONE', #8675, #4780, #7871, .T. ) ;
#4593=CARTESIAN_POINT ( 'NONE',  ( 2.449293598294706513E-15, -20.00000000000000000, -9.999999999999994671 ) ) ;
#4601=CARTESIAN_POINT ( 'NONE',  ( 2.449293598294706513E-15, -20.00000000000000000, -8.999999999999998224 ) ) ;
#4605=FACE_OUTER_BOUND ( 'NONE', #1032, .T. ) ;
#4620=EDGE_CURVE ( 'NONE', #10162, #6905, #576, .T. ) ;
#4621=DIRECTION ( 'NONE',  ( -4.082155997157844188E-16, 1.000000000000000000, 0.000000000000000000 ) ) ;
#4643=VERTEX_POINT ( 'NONE', #8486 ) ;
#4653=CYLINDRICAL_SURFACE ( 'NONE', #13272, 2.149999999999999023 ) ;
#4663=AXIS2_PLACEMENT_3D ( 'NONE', #12635, #250, #10560 ) ;
#4686=AXIS2_PLACEMENT_3D ( 'NONE', #8339, #12471, #13494 ) ;
#4694=ORIENTED_EDGE ( 'NONE', *, *, #623, .T. ) ;
#4714=ORIENTED_EDGE ( 'NONE', *, *, #12713, .T. ) ;
#4717=DIRECTION ( 'NONE',  ( -1.000000000000000000, 1.734723475976806848E-16, 0.000000000000000000 ) ) ;
#4725=FACE_OUTER_BOUND ( 'NONE', #4450, .T. ) ;
#4739=DIRECTION ( 'NONE',  ( -1.000000000000000000, 0.000000000000000000, 0.000000000000000000 ) ) ;
#4750=CARTESIAN_POINT ( 'NONE',  ( 0.8816464618332836567, -24.71833652004169934, 9.999999999999998224 ) ) ;
#4759=EDGE_CURVE ( 'NONE', #7327, #2789, #8724, .T. ) ;
#4780=VERTEX_POINT ( 'NONE', #7248 ) ;
#4784=LINE ( 'NONE', #13134, #4214 ) ;
#4799=DIRECTION ( 'NONE',  ( -0.7779254092217071648, -0.6283566325640553840, 0.000000000000000000 ) ) ;
#4809=DIRECTION ( 'NONE',  ( -1.000000000000000000, 0.000000000000000000, 0.000000000000000000 ) ) ;
#4835=VECTOR ( 'NONE', #2437, 1000.000000000000000 ) ;
#4845=AXIS2_PLACEMENT_3D ( 'NONE', #7274, #11557, #13540 ) ;
#4852=SHAPE_REPRESENTATION_RELATIONSHIP ( 'NONE' , 'NONE' ,  #11036, #12751 ) ;
#4877=MECHANICAL_DESIGN_GEOMETRIC_PRESENTATION_REPRESENTATION('',(#9),#229);
#4886=ORIENTED_EDGE ( 'NONE', *, *, #7173, .F. ) ;
#4887=VERTEX_POINT ( 'NONE', #2936 ) ;
#4906=LINE ( 'NONE', #3718, #12469 ) ;
#4909=CIRCLE ( 'NONE', #10420, 5.000000000000000888 ) ;
#4925=PLANE ( 'NONE',  #9241 ) ;
#4933=CARTESIAN_POINT ( 'NONE',  ( 1.171083334267915221, -24.65495046420793201, 9.000000000000000000 ) ) ;
#4938=ORIENTED_EDGE ( 'NONE', *, *, #12761, .T. ) ;
#4950=DIRECTION ( 'NONE',  ( 9.710251638871371392E-17, 5.969973981896233748E-17, 1.000000000000000000 ) ) ;
#4957=ORIENTED_EDGE ( 'NONE', *, *, #910, .F. ) ;
#4962=DIRECTION ( 'NONE',  ( 9.710251638871371392E-17, 5.969973981896233748E-17, 1.000000000000000000 ) ) ;
#4972=AXIS2_PLACEMENT_3D ( 'NONE', #10561, #5323, #9529 ) ;
#4973=ORIENTED_EDGE ( 'NONE', *, *, #9143, .T. ) ;
#4975=CIRCLE ( 'NONE', #6736, 2.149999999999999023 ) ;
#4979=VERTEX_POINT ( 'NONE', #11435 ) ;
#4991=EDGE_LOOP ( 'NONE', ( #10372, #3860, #3957, #13130 ) ) ;
#4993=ORIENTED_EDGE ( 'NONE', *, *, #13346, .T. ) ;
#4995=CARTESIAN_POINT ( 'NONE',  ( 25.00000000000000711, -20.00000000000000000, -23.00000000000000000 ) ) ;
#5008=ORIENTED_EDGE ( 'NONE', *, *, #2290, .T. ) ;
#5024=PLANE ( 'NONE',  #2622 ) ;
#5042=ORIENTED_EDGE ( 'NONE', *, *, #4759, .T. ) ;
#5050=DIRECTION ( 'NONE',  ( -9.858538378746663627E-23, 5.031452844637890958E-23, -1.000000000000000000 ) ) ;
#5056=LINE ( 'NONE', #13460, #7144 ) ;
#5059=ORIENTED_EDGE ( 'NONE', *, *, #7552, .F. ) ;
#5065=DIRECTION ( 'NONE',  ( -0.9768494444668812671, -0.2139279384389642935, 0.000000000000000000 ) ) ;
#5074=AXIS2_PLACEMENT_3D ( 'NONE', #5713, #435, #10193 ) ;
#5079=VERTEX_POINT ( 'NONE', #6276 ) ;
#5102=CARTESIAN_POINT ( 'NONE',  ( 14.14213562373094923, -14.99999999999999112, -20.00000000000000000 ) ) ;
#5106=CIRCLE ( 'NONE', #2432, 5.000000000000000888 ) ;
#5115=ADVANCED_FACE ( 'NONE', ( #10534 ), #5164, .F. ) ;
#5122=LINE ( 'NONE', #12429, #742 ) ;
#5128=DIRECTION ( 'NONE',  ( -1.000000000000000000, 1.734723475976807094E-16, 0.000000000000000000 ) ) ;
#5133=ORIENTED_EDGE ( 'NONE', *, *, #10454, .F. ) ;
#5134=VECTOR ( 'NONE', #8954, 1000.000000000000000 ) ;
#5149=VERTEX_POINT ( 'NONE', #3342 ) ;
#5153=UNCERTAINTY_MEASURE_WITH_UNIT (LENGTH_MEASURE( 1.000000000000000082E-05 ), #4129, 'distance_accuracy_value', 'NONE');
#5164=CYLINDRICAL_SURFACE ( 'NONE', #4026, 2.149999999999999023 ) ;
#5170=ORIENTED_EDGE ( 'NONE', *, *, #12034, .T. ) ;
#5172=ORIENTED_EDGE ( 'NONE', *, *, #11926, .F. ) ;
#5185=VERTEX_POINT ( 'NONE', #10603 ) ;
#5188=EDGE_CURVE ( 'NONE', #331, #9574, #4246, .T. ) ;
#5189=AXIS2_PLACEMENT_3D ( 'NONE', #2578, #6803, #11008 ) ;
#5192=EDGE_CURVE ( 'NONE', #2677, #12170, #11702, .T. ) ;
#5218=DIRECTION ( 'NONE',  ( 0.000000000000000000, 0.000000000000000000, 1.000000000000000000 ) ) ;
#5225=CARTESIAN_POINT ( 'NONE',  ( -22.14999999999999858, -19.99999999999999289, -20.00000000000000000 ) ) ;
#5243=LINE ( 'NONE', #4260, #1175 ) ;
#5257=CARTESIAN_POINT ( 'NONE',  ( 20.00000000000000000, -20.00000000000000000, -20.00000000000000000 ) ) ;
#5258=PLANE ( 'NONE',  #6665 ) ;
#5270=ORIENTED_EDGE ( 'NONE', *, *, #13275, .F. ) ;
#5300=CARTESIAN_POINT ( 'NONE',  ( 2.449293598294706513E-15, -20.00000000000000000, 9.999999999999998224 ) ) ;
#5307=CARTESIAN_POINT ( 'NONE',  ( 1.219878473194462964, -24.84890673354692936, 15.00000000000000355 ) ) ;
#5318=ORIENTED_EDGE ( 'NONE', *, *, #4567, .F. ) ;
#5323=DIRECTION ( 'NONE',  ( 0.000000000000000000, 0.000000000000000000, -1.000000000000000000 ) ) ;
#5331=CIRCLE ( 'NONE', #13029, 4.800000000000000711 ) ;
#5338=DIRECTION ( 'NONE',  ( -0.000000000000000000, -0.000000000000000000, -1.000000000000000000 ) ) ;
#5347=VECTOR ( 'NONE', #7565, 1000.000000000000000 ) ;
#5349=ADVANCED_FACE ( 'NONE', ( #12050 ), #5766, .F. ) ;
#5363=ADVANCED_FACE ( 'NONE', ( #11773 ), #4653, .F. ) ;
#5379=DIRECTION ( 'NONE',  ( -0.9768494444668813781, -0.2139279384389642935, 1.428280402115105433E-22 ) ) ;
#5385=VECTOR ( 'NONE', #6616, 1000.000000000000000 ) ;
#5389=EDGE_CURVE ( 'NONE', #12172, #12511, #4079, .T. ) ;
#5419=ORIENTED_EDGE ( 'NONE', *, *, #6395, .F. ) ;
#5425=EDGE_CURVE ( 'NONE', #9171, #12678, #9098, .T. ) ;
#5438=ORIENTED_EDGE ( 'NONE', *, *, #8889, .F. ) ;
#5455=ORIENTED_EDGE ( 'NONE', *, *, #10264, .T. ) ;
#5475=CARTESIAN_POINT ( 'NONE',  ( 1.267864665251833278E-11, -20.00000000000000000, 9.000000000000000000 ) ) ;
#5481=ORIENTED_EDGE ( 'NONE', *, *, #11322, .T. ) ;
#5484=CARTESIAN_POINT ( 'NONE',  ( 3.734041964264196434, -16.98388816369253362, -8.999999999999996447 ) ) ;
#5531=CIRCLE ( 'NONE', #1988, 5.000000000000000888 ) ;
#5545=VERTEX_POINT ( 'NONE', #8635 ) ;
#5551=( NAMED_UNIT ( * ) SI_UNIT ( $, .STERADIAN. ) SOLID_ANGLE_UNIT ( ) );
#5557=AXIS2_PLACEMENT_3D ( 'NONE', #3705, #13031, #5866 ) ;
#5558=DIRECTION ( 'NONE',  ( 1.000000000000000000, -1.734723475976807341E-16, 0.000000000000000000 ) ) ;
#5559=CARTESIAN_POINT ( 'NONE',  ( 3.260336594487419859, -23.79080536174652494, -9.999999999999994671 ) ) ;
#5570=DIRECTION ( 'NONE',  ( -9.710251638871371392E-17, -5.969973981896233748E-17, -1.000000000000000000 ) ) ;
#5603=EDGE_CURVE ( 'NONE', #2789, #2711, #10833, .T. ) ;
#5616=ORIENTED_EDGE ( 'NONE', *, *, #7461, .T. ) ;
#5630=VECTOR ( 'NONE', #9332, 1000.000000000000000 ) ;
#5662=LINE ( 'NONE', #6505, #7511 ) ;
#5685=ORIENTED_EDGE ( 'NONE', *, *, #12292, .T. ) ;
#5686=ORIENTED_EDGE ( 'NONE', *, *, #6210, .T. ) ;
#5701=EDGE_CURVE ( 'NONE', #12678, #757, #3502, .T. ) ;
#5710=AXIS2_PLACEMENT_3D ( 'NONE', #3944, #13330, #13398 ) ;
#5713=CARTESIAN_POINT ( 'NONE',  ( 0.8816464618332836567, -24.71833652004169934, 9.999999999999998224 ) ) ;
#5724=CARTESIAN_POINT ( 'NONE',  ( -20.00000000000000000, -19.99999999999999289, -23.00000000000000000 ) ) ;
#5733=AXIS2_PLACEMENT_3D ( 'NONE', #6951, #5918, #12198 ) ;
#5744=DIRECTION ( 'NONE',  ( 9.858538378746663627E-23, -5.031452844637890958E-23, 1.000000000000000000 ) ) ;
#5751=EDGE_LOOP ( 'NONE', ( #12578, #9469, #9453, #4431, #9188, #2556, #12003, #3500 ) ) ;
#5760=FILL_AREA_STYLE ('',( #8734 ) ) ;
#5766=PLANE ( 'NONE',  #12835 ) ;
#5775=CARTESIAN_POINT ( 'NONE',  ( -14.14213562373094568, -25.00000000000000000, -20.00000000000000000 ) ) ;
#5785=MANIFOLD_SOLID_BREP ( 'M4 Clearance Hole1', #2950 ) ;
#5815=VECTOR ( 'NONE', #1102, 1000.000000000000000 ) ;
#5824=ORIENTED_EDGE ( 'NONE', *, *, #3992, .F. ) ;
#5828=CARTESIAN_POINT ( 'NONE',  ( 0.000000000000000000, 0.000000000000000000, 0.000000000000000000 ) ) ;
#5833=DIRECTION ( 'NONE',  ( -0.7779254092217071648, -0.6283566325640553840, 0.000000000000000000 ) ) ;
#5835=CYLINDRICAL_SURFACE ( 'NONE', #13071, 4.799999999999999822 ) ;
#5837=ORIENTED_EDGE ( 'NONE', *, *, #360, .F. ) ;
#5843=AXIS2_PLACEMENT_3D ( 'NONE', #12475, #11440, #13497 ) ;
#5852=DIRECTION ( 'NONE',  ( -0.000000000000000000, -0.000000000000000000, -1.000000000000000000 ) ) ;
#5856=LINE ( 'NONE', #1678, #4512 ) ;
#5864=VECTOR ( 'NONE', #3386, 1000.000000000000000 ) ;
#5866=DIRECTION ( 'NONE',  ( -1.000000000000000000, 0.000000000000000000, 0.000000000000000000 ) ) ;
#5876=CARTESIAN_POINT ( 'NONE',  ( 1.000000000000002442, -20.00000000000000000, -9.000000000000001776 ) ) ;
#5888=VERTEX_POINT ( 'NONE', #3844 ) ;
#5890=VERTEX_POINT ( 'NONE', #7028 ) ;
#5891=AXIS2_PLACEMENT_3D ( 'NONE', #1745, #4950, #2583 ) ;
#5892=VERTEX_POINT ( 'NONE', #713 ) ;
#5905=ORIENTED_EDGE ( 'NONE', *, *, #3479, .T. ) ;
#5906=EDGE_LOOP ( 'NONE', ( #1170, #11863, #4353, #13621, #2400 ) ) ;
#5908=ORIENTED_EDGE ( 'NONE', *, *, #3602, .F. ) ;
#5918=DIRECTION ( 'NONE',  ( -0.000000000000000000, -0.000000000000000000, -1.000000000000000000 ) ) ;
#5935=CARTESIAN_POINT ( 'NONE',  ( -1.000000000000000000, -14.00000000000000000, 8.999999999999998224 ) ) ;
#5965=CARTESIAN_POINT ( 'NONE',  ( -14.14213562373094568, -14.99999999999998757, -20.00000000000000000 ) ) ;
#6000=AXIS2_PLACEMENT_3D ( 'NONE', #3980, #2949, #4128 ) ;
#6014=ORIENTED_EDGE ( 'NONE', *, *, #7461, .F. ) ;
#6022=LINE ( 'NONE', #800, #9160 ) ;
#6036=ORIENTED_EDGE ( 'NONE', *, *, #7625, .T. ) ;
#6054=AXIS2_PLACEMENT_3D ( 'NONE', #2813, #6399, #1106 ) ;
#6058=ORIENTED_EDGE ( 'NONE', *, *, #706, .F. ) ;
#6059=CARTESIAN_POINT ( 'NONE',  ( 2.449293598294706513E-15, -20.00000000000000000, -23.00000000000000000 ) ) ;
#6065=DIRECTION ( 'NONE',  ( 0.6040472319084893016, -0.7969485188038759604, -1.107688701425240097E-17 ) ) ;
#6070=VECTOR ( 'NONE', #7025, 1000.000000000000000 ) ;
#6071=EDGE_LOOP ( 'NONE', ( #6935, #5685 ) ) ;
#6072=EDGE_CURVE ( 'NONE', #12234, #3300, #9914, .T. ) ;
#6075=ORIENTED_EDGE ( 'NONE', *, *, #13206, .T. ) ;
#6098=ADVANCED_FACE ( 'NONE', ( #11998 ), #10881, .T. ) ;
#6104=CARTESIAN_POINT ( 'NONE',  ( 20.00000000000000000, -25.00000000000000711, -20.00000000000000000 ) ) ;
#6107=VERTEX_POINT ( 'NONE', #4392 ) ;
#6112=PLANE ( 'NONE',  #8852 ) ;
#6121=EDGE_LOOP ( 'NONE', ( #5905, #7222, #12939, #2347 ) ) ;
#6143=ORIENTED_EDGE ( 'NONE', *, *, #13179, .T. ) ;
#6146=CARTESIAN_POINT ( 'NONE',  ( 1.000000000000000444, -15.10102051443364246, 15.00000000000000355 ) ) ;
#6158=DIRECTION ( 'NONE',  ( 1.000000000000000000, -1.734723475976807341E-16, 0.000000000000000000 ) ) ;
#6166=ADVANCED_FACE ( 'NONE', ( #6748 ), #1467, .F. ) ;
#6174=ADVANCED_FACE ( 'NONE', ( #8955 ), #3901, .F. ) ;
#6190=ORIENTED_EDGE ( 'NONE', *, *, #9145, .T. ) ;
#6194=VECTOR ( 'NONE', #13119, 999.9999999999998863 ) ;
#6200=ADVANCED_FACE ( 'NONE', ( #13426 ), #5024, .F. ) ;
#6209=LINE ( 'NONE', #10608, #963 ) ;
#6210=EDGE_CURVE ( 'NONE', #10817, #4979, #3954, .T. ) ;
#6214=ORIENTED_EDGE ( 'NONE', *, *, #1611, .F. ) ;
#6224=AXIS2_PLACEMENT_3D ( 'NONE', #8646, #10912, #1360 ) ;
#6233=AXIS2_PLACEMENT_3D ( 'NONE', #7050, #2900, #8161 ) ;
#6247=CIRCLE ( 'NONE', #7108, 4.799999999999999822 ) ;
#6276=CARTESIAN_POINT ( 'NONE',  ( -4.999999999999998224, -20.00000000000000000, -8.999999999999998224 ) ) ;
#6284=DIRECTION ( 'NONE',  ( -9.858538378746663627E-23, 5.031452844637890958E-23, -1.000000000000000000 ) ) ;
#6301=CARTESIAN_POINT ( 'NONE',  ( 2.449293598294706513E-15, -20.00000000000000000, -20.00000000000000000 ) ) ;
#6303=CYLINDRICAL_SURFACE ( 'NONE', #2521, 5.000000000000007994 ) ;
#6328=ORIENTED_EDGE ( 'NONE', *, *, #5701, .F. ) ;
#6338=CIRCLE ( 'NONE', #1972, 5.000000000000000888 ) ;
#6344=DIRECTION ( 'NONE',  ( -1.000000000000000000, 0.000000000000000000, 0.000000000000000000 ) ) ;
#6367=PLANE ( 'NONE',  #4972 ) ;
#6382=CARTESIAN_POINT ( 'NONE',  ( 2.449293598294706513E-15, -20.00000000000000000, 9.000000000000000000 ) ) ;
#6393=ORIENTED_EDGE ( 'NONE', *, *, #10737, .F. ) ;
#6395=EDGE_CURVE ( 'NONE', #2677, #13245, #1357, .T. ) ;
#6399=DIRECTION ( 'NONE',  ( 0.000000000000000000, 0.000000000000000000, -1.000000000000000000 ) ) ;
#6411=ORIENTED_EDGE ( 'NONE', *, *, #13008, .T. ) ;
#6412=DIRECTION ( 'NONE',  ( 0.000000000000000000, 0.000000000000000000, -1.000000000000000000 ) ) ;
#6414=CARTESIAN_POINT ( 'NONE',  ( -19.99999999999999289, -14.99999999999998579, -23.00000000000000000 ) ) ;
#6430=AXIS2_PLACEMENT_3D ( 'NONE', #12879, #8549, #12744 ) ;
#6460=EDGE_LOOP ( 'NONE', ( #10337, #4069, #2697, #10247 ) ) ;
#6461=DIRECTION ( 'NONE',  ( 9.858538378746663627E-23, -5.031452844637890958E-23, 1.000000000000000000 ) ) ;
#6482=DIRECTION ( 'NONE',  ( -1.000000000000000000, 1.734723475976807094E-16, 0.000000000000000000 ) ) ;
#6487=DIRECTION ( 'NONE',  ( -0.000000000000000000, -0.000000000000000000, -1.000000000000000000 ) ) ;
#6492=CIRCLE ( 'NONE', #12428, 5.000000000000000888 ) ;
#6500=CARTESIAN_POINT ( 'NONE',  ( 1.171083334267915221, -24.65495046420793201, 9.999999999999998224 ) ) ;
#6505=CARTESIAN_POINT ( 'NONE',  ( -0.9999999999999976685, -20.00000000000000000, -9.000000000000001776 ) ) ;
#6516=CARTESIAN_POINT ( 'NONE',  ( -0.9999999999999995559, -15.10102051443364246, 9.000000000000000000 ) ) ;
#6520=VECTOR ( 'NONE', #13221, 1000.000000000000000 ) ;
#6562=FACE_BOUND ( 'NONE', #6071, .T. ) ;
#6572=ORIENTED_EDGE ( 'NONE', *, *, #12713, .F. ) ;
#6616=DIRECTION ( 'NONE',  ( 0.000000000000000000, 0.000000000000000000, 1.000000000000000000 ) ) ;
#6654=EDGE_CURVE ( 'NONE', #9272, #11951, #11560, .T. ) ;
#6665=AXIS2_PLACEMENT_3D ( 'NONE', #8628, #4277, #11544 ) ;
#6673=CIRCLE ( 'NONE', #13270, 15.00000000000000000 ) ;
#6689=ORIENTED_EDGE ( 'NONE', *, *, #9143, .F. ) ;
#6719=AXIS2_PLACEMENT_3D ( 'NONE', #10203, #3085, #8137 ) ;
#6723=ORIENTED_EDGE ( 'NONE', *, *, #9122, .T. ) ;
#6727=DIRECTION ( 'NONE',  ( -1.000000000000000000, 0.000000000000000000, 0.000000000000000000 ) ) ;
#6730=CARTESIAN_POINT ( 'NONE',  ( 2.385244779468109755E-15, -20.00000000000000000, -9.999999999999994671 ) ) ;
#6736=AXIS2_PLACEMENT_3D ( 'NONE', #5257, #8429, #10220 ) ;
#6741=DIRECTION ( 'NONE',  ( -1.000000000000000000, 0.000000000000000000, 0.000000000000000000 ) ) ;
#6748=FACE_OUTER_BOUND ( 'NONE', #1209, .T. ) ;
#6753=EDGE_CURVE ( 'NONE', #12170, #504, #692, .T. ) ;
#6757=DIRECTION ( 'NONE',  ( -0.2439756946365075896, 0.9697813467099857254, 1.610118993450814692E-22 ) ) ;
#6761=CARTESIAN_POINT ( 'NONE',  ( -20.00000000000000000, -19.99999999999999289, -23.00000000000000000 ) ) ;
#6763=CYLINDRICAL_SURFACE ( 'NONE', #13229, 4.800000000000000711 ) ;
#6770=DIRECTION ( 'NONE',  ( 0.000000000000000000, 0.000000000000000000, -1.000000000000000000 ) ) ;
#6791=SURFACE_STYLE_USAGE ( .BOTH. , #2562 ) ;
#6797=DIRECTION ( 'NONE',  ( -1.000000000000000000, 0.000000000000000000, 0.000000000000000000 ) ) ;
#6800=VERTEX_POINT ( 'NONE', #1084 ) ;
#6803=DIRECTION ( 'NONE',  ( 9.858538378746663627E-23, -5.031452844637890958E-23, 1.000000000000000000 ) ) ;
#6808=ADVANCED_FACE ( 'NONE', ( #12584 ), #10375, .T. ) ;
#6814=DIRECTION ( 'NONE',  ( -1.000000000000000000, 1.734723475976807094E-16, 0.000000000000000000 ) ) ;
#6821=DIRECTION ( 'NONE',  ( 0.1836763462126260738, -0.9829867750086873635, -1.521953536530129477E-22 ) ) ;
#6825=AXIS2_PLACEMENT_3D ( 'NONE', #781, #1828, #1899 ) ;
#6834=DIRECTION ( 'NONE',  ( -4.082155997157844188E-16, 1.000000000000000000, 0.000000000000000000 ) ) ;
#6836=ORIENTED_EDGE ( 'NONE', *, *, #849, .F. ) ;
#6852=ORIENTED_EDGE ( 'NONE', *, *, #11322, .F. ) ;
#6853=CARTESIAN_POINT ( 'NONE',  ( 20.00000000000000000, -25.00000000000000711, -23.00000000000000000 ) ) ;
#6869=ORIENTED_EDGE ( 'NONE', *, *, #3560, .T. ) ;
#6889=CYLINDRICAL_SURFACE ( 'NONE', #9251, 5.000000000000000888 ) ;
#6894=LINE ( 'NONE', #11101, #683 ) ;
#6905=VERTEX_POINT ( 'NONE', #13301 ) ;
#6922=EDGE_LOOP ( 'NONE', ( #8065, #13609, #10180, #6014 ) ) ;
#6932=CARTESIAN_POINT ( 'NONE',  ( -20.00000000000000000, -25.00000000000000000, -23.00000000000000000 ) ) ;
#6935=ORIENTED_EDGE ( 'NONE', *, *, #11542, .T. ) ;
#6940=LINE ( 'NONE', #1388, #10699 ) ;
#6941=AXIS2_PLACEMENT_3D ( 'NONE', #5300, #7165, #6344 ) ;
#6942=CARTESIAN_POINT ( 'NONE',  ( 2.449293598294706513E-15, -20.00000000000000000, -23.00000000000000000 ) ) ;
#6951=CARTESIAN_POINT ( 'NONE',  ( -20.00000000000000000, -19.99999999999999289, -23.00000000000000000 ) ) ;
#6976=VERTEX_POINT ( 'NONE', #381 ) ;
#6997=DIRECTION ( 'NONE',  ( -1.000000000000000000, 0.000000000000000000, 0.000000000000000000 ) ) ;
#7014=CARTESIAN_POINT ( 'NONE',  ( 2.449293598294706513E-15, -20.00000000000000000, -20.00000000000000000 ) ) ;
#7025=DIRECTION ( 'NONE',  ( -0.000000000000000000, -0.000000000000000000, -1.000000000000000000 ) ) ;
#7028=CARTESIAN_POINT ( 'NONE',  ( -19.99999999999999289, -14.99999999999998579, -20.00000000000000000 ) ) ;
#7043=EDGE_LOOP ( 'NONE', ( #8028, #12374, #5008, #3218 ) ) ;
#7050=CARTESIAN_POINT ( 'NONE',  ( 2.449293598294706513E-15, -20.00000000000000000, -50.00000000000000000 ) ) ;
#7054=CARTESIAN_POINT ( 'NONE',  ( 2.449293598294706513E-15, -20.00000000000000000, -8.999999999999998224 ) ) ;
#7055=CARTESIAN_POINT ( 'NONE',  ( 2.449293598294706513E-15, -20.00000000000000000, 9.999999999999998224 ) ) ;
#7057=EDGE_LOOP ( 'NONE', ( #8438, #6689, #181, #7412 ) ) ;
#7071=ADVANCED_FACE ( 'NONE', ( #8497, #12895 ), #5258, .T. ) ;
#7077=CARTESIAN_POINT ( 'NONE',  ( 20.00000000000000000, -14.99999999999999289, -23.00000000000000000 ) ) ;
#7108=AXIS2_PLACEMENT_3D ( 'NONE', #12394, #7155, #4799 ) ;
#7110=ORIENTED_EDGE ( 'NONE', *, *, #2427, .T. ) ;
#7116=DIRECTION ( 'NONE',  ( -1.000000000000000000, 0.000000000000000000, 0.000000000000000000 ) ) ;
#7135=ADVANCED_FACE ( 'NONE', ( #2188 ), #4208, .F. ) ;
#7144=VECTOR ( 'NONE', #4009, 1000.000000000000000 ) ;
#7150=AXIS2_PLACEMENT_3D ( 'NONE', #12414, #8211, #714 ) ;
#7152=ORIENTED_EDGE ( 'NONE', *, *, #7625, .F. ) ;
#7155=DIRECTION ( 'NONE',  ( 9.710251638871371392E-17, 5.969973981896233748E-17, 1.000000000000000000 ) ) ;
#7156=PRODUCT_CONTEXT ( 'NONE', #3544, 'mechanical' ) ;
#7165=DIRECTION ( 'NONE',  ( -9.858538378746663627E-23, 5.031452844637890958E-23, -1.000000000000000000 ) ) ;
#7169=ORIENTED_EDGE ( 'NONE', *, *, #3769, .F. ) ;
#7173=EDGE_CURVE ( 'NONE', #12840, #12234, #11026, .T. ) ;
#7176=CYLINDRICAL_SURFACE ( 'NONE', #7150, 4.799999999999999822 ) ;
#7184=EDGE_CURVE ( 'NONE', #5888, #6976, #8832, .T. ) ;
#7191=DIRECTION ( 'NONE',  ( -1.734723475976807341E-16, -1.000000000000000000, 0.000000000000000000 ) ) ;
#7205=ADVANCED_FACE ( 'NONE', ( #9991 ), #12958, .T. ) ;
#7222=ORIENTED_EDGE ( 'NONE', *, *, #3233, .T. ) ;
#7241=ORIENTED_EDGE ( 'NONE', *, *, #12236, .T. ) ;
#7244=LINE ( 'NONE', #6146, #6070 ) ;
#7248=CARTESIAN_POINT ( 'NONE',  ( 1.000000000000000000, -14.00000000000000000, 8.999999999999998224 ) ) ;
#7256=CARTESIAN_POINT ( 'NONE',  ( 20.00000000000000000, -20.00000000000000000, -23.00000000000000000 ) ) ;
#7273=EDGE_CURVE ( 'NONE', #1489, #5890, #10626, .T. ) ;
#7274=CARTESIAN_POINT ( 'NONE',  ( 2.449293598294706513E-15, -20.00000000000000000, -50.00000000000000000 ) ) ;
#7284=DIRECTION ( 'NONE',  ( -0.000000000000000000, -0.000000000000000000, -1.000000000000000000 ) ) ;
#7292=EDGE_CURVE ( 'NONE', #3770, #10906, #4784, .T. ) ;
#7314=ORIENTED_EDGE ( 'NONE', *, *, #3817, .F. ) ;
#7322=DIRECTION ( 'NONE',  ( -1.000000000000000000, 0.000000000000000000, 0.000000000000000000 ) ) ;
#7327=VERTEX_POINT ( 'NONE', #2526 ) ;
#7335=AXIS2_PLACEMENT_3D ( 'NONE', #3644, #445, #11099 ) ;
#7337=CARTESIAN_POINT ( 'NONE',  ( 2.449293598294706513E-15, -20.00000000000000000, 9.000000000000000000 ) ) ;
#7347=FACE_OUTER_BOUND ( 'NONE', #3517, .T. ) ;
#7360=EDGE_LOOP ( 'NONE', ( #7152, #131, #1334, #9422 ) ) ;
#7375=PLANE ( 'NONE',  #2746 ) ;
#7384=CYLINDRICAL_SURFACE ( 'NONE', #1088, 5.000000000000000888 ) ;
#7394=CARTESIAN_POINT ( 'NONE',  ( 20.00000000000000000, -14.99999999999999289, -23.00000000000000000 ) ) ;
#7405=CARTESIAN_POINT ( 'NONE',  ( 3.129923130707922496, -23.63917314727666152, -9.999999999999994671 ) ) ;
#7412=ORIENTED_EDGE ( 'NONE', *, *, #2346, .T. ) ;
#7424=ORIENTED_EDGE ( 'NONE', *, *, #8680, .F. ) ;
#7425=ORIENTED_EDGE ( 'NONE', *, *, #11433, .T. ) ;
#7426=LINE ( 'NONE', #10593, #5815 ) ;
#7458=ADVANCED_FACE ( 'NONE', ( #13436 ), #3018, .T. ) ;
#7461=EDGE_CURVE ( 'NONE', #12172, #651, #10545, .T. ) ;
#7481=CARTESIAN_POINT ( 'NONE',  ( 0.9183817310753817909, -24.91493387504115020, 9.000000000000000000 ) ) ;
#7486=ORIENTED_EDGE ( 'NONE', *, *, #260, .T. ) ;
#7491=ADVANCED_FACE ( 'NONE', ( #2169 ), #2042, .T. ) ;
#7507=LINE ( 'NONE', #11715, #8644 ) ;
#7511=VECTOR ( 'NONE', #4621, 1000.000000000000000 ) ;
#7514=CARTESIAN_POINT ( 'NONE',  ( 2.385244779468109755E-15, -20.00000000000000000, -9.999999999999994671 ) ) ;
#7519=EDGE_CURVE ( 'NONE', #13554, #12511, #11593, .T. ) ;
#7525=EDGE_CURVE ( 'NONE', #9611, #690, #4325, .T. ) ;
#7548=AXIS2_PLACEMENT_3D ( 'NONE', #7514, #9720, #9852 ) ;
#7552=EDGE_CURVE ( 'NONE', #10817, #10955, #7507, .T. ) ;
#7556=DIRECTION ( 'NONE',  ( -0.000000000000000000, -0.000000000000000000, -1.000000000000000000 ) ) ;
#7565=DIRECTION ( 'NONE',  ( -0.000000000000000000, -0.000000000000000000, -1.000000000000000000 ) ) ;
#7575=CARTESIAN_POINT ( 'NONE',  ( 1.171083334267915221, -24.65495046420793201, 9.999999999999998224 ) ) ;
#7580=FACE_OUTER_BOUND ( 'NONE', #1264, .T. ) ;
#7589=PRODUCT_DEFINITION_CONTEXT ( 'detailed design', #13418, 'design' ) ;
#7605=ORIENTED_EDGE ( 'NONE', *, *, #12348, .T. ) ;
#7616=VECTOR ( 'NONE', #10280, 1000.000000000000000 ) ;
#7625=EDGE_CURVE ( 'NONE', #2771, #5545, #11992, .T. ) ;
#7626=CARTESIAN_POINT ( 'NONE',  ( 2.449293598294706513E-15, -20.00000000000000000, 9.000000000000000000 ) ) ;
#7638=ORIENTED_EDGE ( 'NONE', *, *, #2719, .F. ) ;
#7675=CARTESIAN_POINT ( 'NONE',  ( 5.000000000000003553, -20.00000000000000000, 15.00000000000000355 ) ) ;
#7676=DIRECTION ( 'NONE',  ( 1.000000000000000000, 0.000000000000000000, 0.000000000000000000 ) ) ;
#7685=ORIENTED_EDGE ( 'NONE', *, *, #1708, .T. ) ;
#7696=CIRCLE ( 'NONE', #12326, 5.000000000000007994 ) ;
#7701=EDGE_CURVE ( 'NONE', #9611, #8761, #6673, .T. ) ;
#7703=FACE_OUTER_BOUND ( 'NONE', #2181, .T. ) ;
#7711=VECTOR ( 'NONE', #1204, 1000.000000000000000 ) ;
#7724=ORIENTED_EDGE ( 'NONE', *, *, #13275, .T. ) ;
#7743=ORIENTED_EDGE ( 'NONE', *, *, #11147, .F. ) ;
#7744=ORIENTED_EDGE ( 'NONE', *, *, #7807, .T. ) ;
#7746=ORIENTED_EDGE ( 'NONE', *, *, #7292, .T. ) ;
#7761=LINE ( 'NONE', #5484, #10508 ) ;
#7762=CARTESIAN_POINT ( 'NONE',  ( -4.999999999999998224, -20.00000000000000000, 15.00000000000000355 ) ) ;
#7769=ADVANCED_FACE ( 'NONE', ( #11150 ), #8190, .T. ) ;
#7775=DIRECTION ( 'NONE',  ( 4.082155997157843695E-16, -1.000000000000000000, 0.000000000000000000 ) ) ;
#7790=CARTESIAN_POINT ( 'NONE',  ( 20.00000000000000000, -25.00000000000000711, -23.00000000000000000 ) ) ;
#7807=EDGE_CURVE ( 'NONE', #2711, #3301, #6247, .T. ) ;
#7812=DIRECTION ( 'NONE',  ( -4.082155997157844188E-16, 1.000000000000000000, 0.000000000000000000 ) ) ;
#7837=AXIS2_PLACEMENT_3D ( 'NONE', #12269, #3837, #4809 ) ;
#7871=LINE ( 'NONE', #5935, #7616 ) ;
#7899=CARTESIAN_POINT ( 'NONE',  ( 1.267864665251833278E-11, -20.00000000000000000, 9.000000000000000000 ) ) ;
#7915=AXIS2_PLACEMENT_3D ( 'NONE', #12858, #217, #4436 ) ;
#7925=CARTESIAN_POINT ( 'NONE',  ( 2.449293598294706513E-15, -20.00000000000000000, 15.00000000000000355 ) ) ;
#7954=DIRECTION ( 'NONE',  ( -1.000000000000000000, 0.000000000000000000, 0.000000000000000000 ) ) ;
#7964=DIRECTION ( 'NONE',  ( -0.000000000000000000, -0.000000000000000000, -1.000000000000000000 ) ) ;
#8019=FACE_OUTER_BOUND ( 'NONE', #1574, .T. ) ;
#8022=CARTESIAN_POINT ( 'NONE',  ( 2.449293598294706513E-15, -20.00000000000000000, -9.999999999999994671 ) ) ;
#8028=ORIENTED_EDGE ( 'NONE', *, *, #2427, .F. ) ;
#8029=LINE ( 'NONE', #11845, #10781 ) ;
#8046=ORIENTED_EDGE ( 'NONE', *, *, #7525, .F. ) ;
#8048=LINE ( 'NONE', #12258, #2298 ) ;
#8065=ORIENTED_EDGE ( 'NONE', *, *, #5389, .T. ) ;
#8100=ORIENTED_EDGE ( 'NONE', *, *, #849, .T. ) ;
#8132=EDGE_CURVE ( 'NONE', #3300, #5185, #8217, .T. ) ;
#8137=DIRECTION ( 'NONE',  ( -1.000000000000000000, 0.000000000000000000, 0.000000000000000000 ) ) ;
#8146=AXIS2_PLACEMENT_3D ( 'NONE', #7256, #1844, #1916 ) ;
#8161=DIRECTION ( 'NONE',  ( 1.000000000000000000, 0.000000000000000000, 0.000000000000000000 ) ) ;
#8180=CARTESIAN_POINT ( 'NONE',  ( 2.449293598294706513E-15, -20.00000000000000000, 15.00000000000000355 ) ) ;
#8190=PLANE ( 'NONE',  #12832 ) ;
#8211=DIRECTION ( 'NONE',  ( -9.710251638871371392E-17, -5.969973981896233748E-17, -1.000000000000000000 ) ) ;
#8217=CIRCLE ( 'NONE', #2234, 5.000000000000000888 ) ;
#8251=DIRECTION ( 'NONE',  ( 1.000000000000000000, 0.000000000000000000, 0.000000000000000000 ) ) ;
#8257=ORIENTED_EDGE ( 'NONE', *, *, #8680, .T. ) ;
#8259=DIRECTION ( 'NONE',  ( -0.000000000000000000, -0.000000000000000000, -1.000000000000000000 ) ) ;
#8272=CIRCLE ( 'NONE', #3179, 4.799999999999999822 ) ;
#8290=ORIENTED_EDGE ( 'NONE', *, *, #3246, .F. ) ;
#8298=DIRECTION ( 'NONE',  ( -0.000000000000000000, -0.000000000000000000, -1.000000000000000000 ) ) ;
#8313=CARTESIAN_POINT ( 'NONE',  ( 20.00000000000000000, -20.00000000000000000, -23.00000000000000000 ) ) ;
#8320=LINE ( 'NONE', #9215, #9984 ) ;
#8327=UNCERTAINTY_MEASURE_WITH_UNIT (LENGTH_MEASURE( 1.000000000000000082E-05 ), #1931, 'distance_accuracy_value', 'NONE');
#8339=CARTESIAN_POINT ( 'NONE',  ( 20.00000000000000000, -20.00000000000000000, -20.00000000000000000 ) ) ;
#8344=ADVANCED_FACE ( 'NONE', ( #1868 ), #813, .F. ) ;
#8345=CARTESIAN_POINT ( 'NONE',  ( 5.000000000000003553, -20.00000000000000000, 9.000000000000000000 ) ) ;
#8367=CARTESIAN_POINT ( 'NONE',  ( 5.000000000000003553, -20.00000000000000000, 9.999999999999998224 ) ) ;
#8370=ADVANCED_FACE ( 'NONE', ( #2912, #11346 ), #6112, .T. ) ;
#8399=EDGE_CURVE ( 'NONE', #12971, #8775, #5331, .T. ) ;
#8426=ORIENTED_EDGE ( 'NONE', *, *, #1697, .F. ) ;
#8427=ORIENTED_EDGE ( 'NONE', *, *, #13444, .F. ) ;
#8429=DIRECTION ( 'NONE',  ( 0.000000000000000000, 0.000000000000000000, -1.000000000000000000 ) ) ;
#8431=DIRECTION ( 'NONE',  ( 1.000000000000000000, 0.000000000000000000, 0.000000000000000000 ) ) ;
#8438=ORIENTED_EDGE ( 'NONE', *, *, #4620, .F. ) ;
#8442=CARTESIAN_POINT ( 'NONE',  ( 0.000000000000000000, 0.000000000000000000, -9.000000000000001776 ) ) ;
#8449=CARTESIAN_POINT ( 'NONE',  ( 3.734041964264196878, -16.98388816369253362, -9.999999999999994671 ) ) ;
#8452=EDGE_LOOP ( 'NONE', ( #7638, #6411, #538, #1473 ) ) ;
#8460=VECTOR ( 'NONE', #5128, 1000.000000000000000 ) ;
#8464=CARTESIAN_POINT ( 'NONE',  ( 5.000000000000003553, -20.00000000000000000, 15.00000000000000355 ) ) ;
#8475=EDGE_CURVE ( 'NONE', #3147, #347, #5106, .T. ) ;
#8477=DIRECTION ( 'NONE',  ( -1.000000000000000000, 0.000000000000000000, 0.000000000000000000 ) ) ;
#8486=CARTESIAN_POINT ( 'NONE',  ( -4.688877333428352223, -21.02685410450703074, 9.999999999999998224 ) ) ;
#8495=CIRCLE ( 'NONE', #1620, 5.000000000000000888 ) ;
#8497=FACE_BOUND ( 'NONE', #10072, .T. ) ;
#8503=VECTOR ( 'NONE', #8298, 1000.000000000000000 ) ;
#8510=ORIENTED_EDGE ( 'NONE', *, *, #281, .T. ) ;
#8549=DIRECTION ( 'NONE',  ( -0.000000000000000000, -0.000000000000000000, 1.000000000000000000 ) ) ;
#8557=ORIENTED_EDGE ( 'NONE', *, *, #8889, .T. ) ;
#8564=FACE_OUTER_BOUND ( 'NONE', #8452, .T. ) ;
#8572=VERTEX_POINT ( 'NONE', #12444 ) ;
#8575=VECTOR ( 'NONE', #2698, 1000.000000000000000 ) ;
#8587=EDGE_LOOP ( 'NONE', ( #4541, #1434, #12825, #8807 ) ) ;
#8588=DIRECTION ( 'NONE',  ( -9.710251638871371392E-17, -5.969973981896233748E-17, -1.000000000000000000 ) ) ;
#8597=VECTOR ( 'NONE', #1385, 1000.000000000000000 ) ;
#8598=DIRECTION ( 'NONE',  ( -0.000000000000000000, -0.000000000000000000, -1.000000000000000000 ) ) ;
#8600=ADVANCED_FACE ( 'NONE', ( #1492 ), #9677, .T. ) ;
#8610=PLANE ( 'NONE',  #4285 ) ;
#8626=CARTESIAN_POINT ( 'NONE',  ( -4.999999999999998224, -20.00000000000000000, 15.00000000000000355 ) ) ;
#8628=CARTESIAN_POINT ( 'NONE',  ( 20.00000000000000000, -20.00000000000000000, -23.00000000000000000 ) ) ;
#8635=CARTESIAN_POINT ( 'NONE',  ( -17.85000000000000142, -19.99999999999999289, -23.00000000000000000 ) ) ;
#8644=VECTOR ( 'NONE', #9644, 1000.000000000000000 ) ;
#8646=CARTESIAN_POINT ( 'NONE',  ( 2.482347295856823136E-15, -20.00000000000000000, -8.999999999999996447 ) ) ;
#8675=VERTEX_POINT ( 'NONE', #2267 ) ;
#8676=DIRECTION ( 'NONE',  ( -1.000000000000000000, -4.082155997157843695E-16, 0.000000000000000000 ) ) ;
#8680=EDGE_CURVE ( 'NONE', #1421, #5149, #10170, .T. ) ;
#8685=CARTESIAN_POINT ( 'NONE',  ( 1.267864665261691752E-11, -20.00000000000000000, 9.999999999999998224 ) ) ;
#8687=DIRECTION ( 'NONE',  ( -9.710251638871371392E-17, -5.969973981896233748E-17, -1.000000000000000000 ) ) ;
#8718=AXIS2_PLACEMENT_3D ( 'NONE', #3031, #13383, #3927 ) ;
#8724=CIRCLE ( 'NONE', #2088, 5.000000000000000888 ) ;
#8728=ORIENTED_EDGE ( 'NONE', *, *, #4163, .F. ) ;
#8734=FILL_AREA_STYLE_COLOUR ( '', #13458 ) ;
#8735=DIRECTION ( 'NONE',  ( -9.858538378746663627E-23, 5.031452844637890958E-23, -1.000000000000000000 ) ) ;
#8743=ORIENTED_EDGE ( 'NONE', *, *, #11147, .T. ) ;
#8747=DIRECTION ( 'NONE',  ( -1.000000000000000000, 0.000000000000000000, 0.000000000000000000 ) ) ;
#8753=CARTESIAN_POINT ( 'NONE',  ( 1.267864665261691752E-11, -20.00000000000000000, 9.999999999999998224 ) ) ;
#8757=CARTESIAN_POINT ( 'NONE',  ( 3.260336594487421635, -23.79080536174652494, 15.00000000000000355 ) ) ;
#8758=ORIENTED_EDGE ( 'NONE', *, *, #12348, .F. ) ;
#8761=VERTEX_POINT ( 'NONE', #202 ) ;
#8764=DIRECTION ( 'NONE',  ( -9.710251638871371392E-17, -5.969973981896233748E-17, -1.000000000000000000 ) ) ;
#8775=VERTEX_POINT ( 'NONE', #4423 ) ;
#8793=( NAMED_UNIT ( * ) PLANE_ANGLE_UNIT ( ) SI_UNIT ( $, .RADIAN. ) );
#8807=ORIENTED_EDGE ( 'NONE', *, *, #10424, .F. ) ;
#8809=CIRCLE ( 'NONE', #2392, 2.149999999999999023 ) ;
#8823=LINE ( 'NONE', #8757, #5385 ) ;
#8824=ORIENTED_EDGE ( 'NONE', *, *, #6072, .T. ) ;
#8831=PRODUCT_DEFINITION_FORMATION_WITH_SPECIFIED_SOURCE ( 'ANY', '', #1011, .NOT_KNOWN. ) ;
#8832=LINE ( 'NONE', #1546, #1110 ) ;
#8852=AXIS2_PLACEMENT_3D ( 'NONE', #10027, #11202, #13468 ) ;
#8858=EDGE_LOOP ( 'NONE', ( #148, #12235, #8100, #1840 ) ) ;
#8865=SURFACE_STYLE_FILL_AREA ( #5760 ) ;
#8889=EDGE_CURVE ( 'NONE', #3906, #3300, #10009, .T. ) ;
#8934=CARTESIAN_POINT ( 'NONE',  ( 2.449293598294706513E-15, -20.00000000000000000, -50.00000000000000000 ) ) ;
#8935=AXIS2_PLACEMENT_3D ( 'NONE', #6059, #1950, #902 ) ;
#8954=DIRECTION ( 'NONE',  ( -0.000000000000000000, -0.000000000000000000, -1.000000000000000000 ) ) ;
#8955=FACE_OUTER_BOUND ( 'NONE', #3656, .T. ) ;
#9024=ORIENTED_EDGE ( 'NONE', *, *, #7701, .T. ) ;
#9027=EDGE_LOOP ( 'NONE', ( #7743, #150 ) ) ;
#9040=AXIS2_PLACEMENT_3D ( 'NONE', #3280, #8676, #7775 ) ;
#9045=VECTOR ( 'NONE', #10776, 1000.000000000000000 ) ;
#9049=VECTOR ( 'NONE', #12119, 1000.000000000000000 ) ;
#9064=ORIENTED_EDGE ( 'NONE', *, *, #10658, .T. ) ;
#9068=CARTESIAN_POINT ( 'NONE',  ( 20.00000000000000000, -14.99999999999999289, -23.00000000000000000 ) ) ;
#9079=ORIENTED_EDGE ( 'NONE', *, *, #5389, .F. ) ;
#9098=CIRCLE ( 'NONE', #1790, 5.000000000000000888 ) ;
#9101=ORIENTED_EDGE ( 'NONE', *, *, #3742, .T. ) ;
#9117=ORIENTED_EDGE ( 'NONE', *, *, #12236, .F. ) ;
#9122=EDGE_CURVE ( 'NONE', #3301, #6976, #3528, .T. ) ;
#9132=EDGE_LOOP ( 'NONE', ( #9101, #13225, #263, #9202 ) ) ;
#9143=EDGE_CURVE ( 'NONE', #8675, #10162, #13121, .T. ) ;
#9145=EDGE_CURVE ( 'NONE', #8775, #3906, #11479, .T. ) ;
#9150=VERTEX_POINT ( 'NONE', #1293 ) ;
#9160=VECTOR ( 'NONE', #5050, 1000.000000000000000 ) ;
#9171=VERTEX_POINT ( 'NONE', #9679 ) ;
#9188=ORIENTED_EDGE ( 'NONE', *, *, #5603, .F. ) ;
#9202=ORIENTED_EDGE ( 'NONE', *, *, #2185, .T. ) ;
#9215=CARTESIAN_POINT ( 'NONE',  ( 5.000000000000003553, -20.00000000000000000, 15.00000000000000355 ) ) ;
#9222=DIRECTION ( 'NONE',  ( -1.000000000000000000, 1.734723475976807094E-16, 0.000000000000000000 ) ) ;
#9229=CARTESIAN_POINT ( 'NONE',  ( 3.129923130707922496, -23.63917314727666152, -9.999999999999994671 ) ) ;
#9230=DIRECTION ( 'NONE',  ( 0.000000000000000000, 0.000000000000000000, -1.000000000000000000 ) ) ;
#9241=AXIS2_PLACEMENT_3D ( 'NONE', #6853, #12376, #4717 ) ;
#9245=FACE_OUTER_BOUND ( 'NONE', #864, .T. ) ;
#9251=AXIS2_PLACEMENT_3D ( 'NONE', #7925, #9859, #2591 ) ;
#9271=ORIENTED_EDGE ( 'NONE', *, *, #8475, .F. ) ;
#9272=VERTEX_POINT ( 'NONE', #6516 ) ;
#9308=ORIENTED_EDGE ( 'NONE', *, *, #103, .T. ) ;
#9313=( NAMED_UNIT ( * ) SI_UNIT ( $, .STERADIAN. ) SOLID_ANGLE_UNIT ( ) );
#9322=ADVANCED_FACE ( 'NONE', ( #8019 ), #2614, .T. ) ;
#9332=DIRECTION ( 'NONE',  ( 1.000000000000000000, -1.734723475976807341E-16, -0.000000000000000000 ) ) ;
#9345=CIRCLE ( 'NONE', #3380, 4.800000000000000711 ) ;
#9357=ORIENTED_EDGE ( 'NONE', *, *, #13352, .T. ) ;
#9400=DIRECTION ( 'NONE',  ( 0.000000000000000000, 0.000000000000000000, -1.000000000000000000 ) ) ;
#9414=DIRECTION ( 'NONE',  ( -1.000000000000000000, 0.000000000000000000, 0.000000000000000000 ) ) ;
#9422=ORIENTED_EDGE ( 'NONE', *, *, #2529, .T. ) ;
#9427=CARTESIAN_POINT ( 'NONE',  ( 1.171083334267915221, -24.65495046420793201, 9.999999999999998224 ) ) ;
#9453=ORIENTED_EDGE ( 'NONE', *, *, #9122, .F. ) ;
#9454=PRODUCT_DEFINITION ( 'UNKNOWN', '', #8831, #7589 ) ;
#9457=CARTESIAN_POINT ( 'NONE',  ( -20.00000000000000000, -19.99999999999999289, -20.00000000000000000 ) ) ;
#9459=DIRECTION ( 'NONE',  ( -0.000000000000000000, -0.000000000000000000, 1.000000000000000000 ) ) ;
#9462=AXIS2_PLACEMENT_3D ( 'NONE', #2891, #7191, #6158 ) ;
#9469=ORIENTED_EDGE ( 'NONE', *, *, #2290, .F. ) ;
#9515=DIRECTION ( 'NONE',  ( -0.000000000000000000, -0.000000000000000000, -1.000000000000000000 ) ) ;
#9529=DIRECTION ( 'NONE',  ( -1.000000000000000000, 0.000000000000000000, -0.000000000000000000 ) ) ;
#9574=VERTEX_POINT ( 'NONE', #8367 ) ;
#9580=EDGE_CURVE ( 'NONE', #5185, #9272, #5531, .T. ) ;
#9611=VERTEX_POINT ( 'NONE', #10706 ) ;
#9614=CIRCLE ( 'NONE', #6719, 5.000000000000000888 ) ;
#9624=EDGE_LOOP ( 'NONE', ( #13636, #12496, #6190, #179 ) ) ;
#9633=AXIS2_PLACEMENT_3D ( 'NONE', #7014, #9978, #498 ) ;
#9640=CARTESIAN_POINT ( 'NONE',  ( 3.260336594487419859, -23.79080536174652494, -8.999999999999998224 ) ) ;
#9644=DIRECTION ( 'NONE',  ( -0.000000000000000000, -0.000000000000000000, 1.000000000000000000 ) ) ;
#9651=DIRECTION ( 'NONE',  ( -0.9768494444668812671, -0.2139279384389642935, 0.000000000000000000 ) ) ;
#9664=ADVANCED_FACE ( 'NONE', ( #190 ), #6763, .T. ) ;
#9668=DIRECTION ( 'NONE',  ( -0.9768494444668812671, -0.2139279384389642935, 0.000000000000000000 ) ) ;
#9677=CYLINDRICAL_SURFACE ( 'NONE', #2214, 5.000000000000007994 ) ;
#9679=CARTESIAN_POINT ( 'NONE',  ( 1.000000000000000444, -15.10102051443364246, -8.999999999999998224 ) ) ;
#9706=AXIS2_PLACEMENT_3D ( 'NONE', #6730, #3615, #5833 ) ;
#9712=ADVANCED_FACE ( 'NONE', ( #8564 ), #12901, .F. ) ;
#9719=EDGE_CURVE ( 'NONE', #11951, #10162, #5662, .T. ) ;
#9720=DIRECTION ( 'NONE',  ( 9.710251638871371392E-17, 5.969973981896233748E-17, 1.000000000000000000 ) ) ;
#9732=CARTESIAN_POINT ( 'NONE',  ( 25.00000000000000711, -20.00000000000000000, -20.00000000000000000 ) ) ;
#9748=DIRECTION ( 'NONE',  ( -0.000000000000000000, -0.000000000000000000, 1.000000000000000000 ) ) ;
#9756=VECTOR ( 'NONE', #11922, 1000.000000000000000 ) ;
#9769=CARTESIAN_POINT ( 'NONE',  ( 20.00000000000000000, -20.00000000000000000, -23.00000000000000000 ) ) ;
#9775=CARTESIAN_POINT ( 'NONE',  ( -20.00000000000000000, -25.00000000000000000, -23.00000000000000000 ) ) ;
#9777=CARTESIAN_POINT ( 'NONE',  ( 3.020236159542450949, -23.98474259401938014, 15.00000000000000355 ) ) ;
#9783=CYLINDRICAL_SURFACE ( 'NONE', #6430, 5.000000000000007994 ) ;
#9786=CARTESIAN_POINT ( 'NONE',  ( 0.9183817310753816798, -24.91493387504114665, 15.00000000000000355 ) ) ;
#9800=DIRECTION ( 'NONE',  ( 0.000000000000000000, 0.000000000000000000, -1.000000000000000000 ) ) ;
#9807=CIRCLE ( 'NONE', #8935, 15.00000000000000000 ) ;
#9808=ORIENTED_EDGE ( 'NONE', *, *, #4262, .F. ) ;
#9852=DIRECTION ( 'NONE',  ( -0.7779254092217071648, -0.6283566325640553840, 0.000000000000000000 ) ) ;
#9859=DIRECTION ( 'NONE',  ( -0.000000000000000000, -0.000000000000000000, -1.000000000000000000 ) ) ;
#9866=CARTESIAN_POINT ( 'NONE',  ( 2.899426713160750069, -23.82535289025860337, -8.999999999999996447 ) ) ;
#9885=ORIENTED_EDGE ( 'NONE', *, *, #12034, .F. ) ;
#9897=EDGE_CURVE ( 'NONE', #4643, #8775, #12557, .T. ) ;
#9903=ORIENTED_EDGE ( 'NONE', *, *, #3560, .F. ) ;
#9907=CARTESIAN_POINT ( 'NONE',  ( 22.14999999999999858, -20.00000000000000000, -20.00000000000000000 ) ) ;
#9914=LINE ( 'NONE', #9786, #7711 ) ;
#9922=DIRECTION ( 'NONE',  ( -1.000000000000000000, 0.000000000000000000, 0.000000000000000000 ) ) ;
#9930=ADVANCED_FACE ( 'NONE', ( #10482 ), #7384, .T. ) ;
#9969=ORIENTED_EDGE ( 'NONE', *, *, #2529, .F. ) ;
#9975=DIRECTION ( 'NONE',  ( -0.000000000000000000, -0.000000000000000000, -1.000000000000000000 ) ) ;
#9978=DIRECTION ( 'NONE',  ( 0.000000000000000000, 0.000000000000000000, 1.000000000000000000 ) ) ;
#9984=VECTOR ( 'NONE', #7284, 1000.000000000000000 ) ;
#9991=FACE_OUTER_BOUND ( 'NONE', #3265, .T. ) ;
#9994=DIRECTION ( 'NONE',  ( -1.000000000000000000, 0.000000000000000000, 0.000000000000000000 ) ) ;
#9995=VECTOR ( 'NONE', #12095, 1000.000000000000000 ) ;
#10009=LINE ( 'NONE', #13315, #6194 ) ;
#10027=CARTESIAN_POINT ( 'NONE',  ( 20.00000000000000000, -20.00000000000000000, -23.00000000000000000 ) ) ;
#10050=CARTESIAN_POINT ( 'NONE',  ( -4.999999999999998224, -20.00000000000000000, 15.00000000000000355 ) ) ;
#10063=ADVANCED_FACE ( 'NONE', ( #12946 ), #171, .T. ) ;
#10066=ADVANCED_FACE ( 'NONE', ( #7580 ), #9783, .T. ) ;
#10072=EDGE_LOOP ( 'NONE', ( #11095, #6393 ) ) ;
#10073=ORIENTED_EDGE ( 'NONE', *, *, #3170, .F. ) ;
#10092=FACE_OUTER_BOUND ( 'NONE', #1716, .T. ) ;
#10100=DIRECTION ( 'NONE',  ( -9.710251638871371392E-17, -5.969973981896233748E-17, -1.000000000000000000 ) ) ;
#10103=VECTOR ( 'NONE', #6834, 1000.000000000000000 ) ;
#10106=DIRECTION ( 'NONE',  ( -1.000000000000000000, 0.000000000000000000, 0.000000000000000000 ) ) ;
#10162=VERTEX_POINT ( 'NONE', #13559 ) ;
#10164=VERTEX_POINT ( 'NONE', #12532 ) ;
#10166=CARTESIAN_POINT ( 'NONE',  ( -20.00000000000000000, -19.99999999999999289, -20.00000000000000000 ) ) ;
#10170=CIRCLE ( 'NONE', #6224, 4.799999999999999822 ) ;
#10172=DIRECTION ( 'NONE',  ( 9.858538378746663627E-23, -5.031452844637890958E-23, 1.000000000000000000 ) ) ;
#10178=CARTESIAN_POINT ( 'NONE',  ( 1.000000000000000444, -15.10102051443364246, 9.000000000000000000 ) ) ;
#10180=ORIENTED_EDGE ( 'NONE', *, *, #12525, .F. ) ;
#10193=DIRECTION ( 'NONE',  ( 0.1836763462126260182, -0.9829867750086872524, -1.521953536530129242E-22 ) ) ;
#10199=VECTOR ( 'NONE', #1730, 1000.000000000000000 ) ;
#10203=CARTESIAN_POINT ( 'NONE',  ( 2.449293598294706513E-15, -20.00000000000000000, 9.999999999999998224 ) ) ;
#10220=DIRECTION ( 'NONE',  ( -1.000000000000000000, 0.000000000000000000, 0.000000000000000000 ) ) ;
#10239=AXIS2_PLACEMENT_3D ( 'NONE', #5724, #13161, #9922 ) ;
#10247=ORIENTED_EDGE ( 'NONE', *, *, #9897, .F. ) ;
#10252=DIRECTION ( 'NONE',  ( -0.000000000000000000, -0.000000000000000000, 1.000000000000000000 ) ) ;
#10264=EDGE_CURVE ( 'NONE', #10164, #5892, #3470, .T. ) ;
#10267=LINE ( 'NONE', #10050, #6520 ) ;
#10273=ADVANCED_FACE ( 'NONE', ( #12791 ), #283, .T. ) ;
#10280=DIRECTION ( 'NONE',  ( 1.000000000000000000, 0.000000000000000000, 0.000000000000000000 ) ) ;
#10285=ORIENTED_EDGE ( 'NONE', *, *, #3742, .F. ) ;
#10329=CARTESIAN_POINT ( 'NONE',  ( 2.899426713160750069, -23.82535289025860337, -8.999999999999996447 ) ) ;
#10337=ORIENTED_EDGE ( 'NONE', *, *, #11945, .F. ) ;
#10368=LINE ( 'NONE', #6104, #8460 ) ;
#10372=ORIENTED_EDGE ( 'NONE', *, *, #8475, .T. ) ;
#10375=PLANE ( 'NONE',  #13499 ) ;
#10392=LINE ( 'NONE', #3062, #2974 ) ;
#10413=CARTESIAN_POINT ( 'NONE',  ( -4.688877333428353111, -21.02685410450703074, 9.999999999999998224 ) ) ;
#10420=AXIS2_PLACEMENT_3D ( 'NONE', #4601, #8687, #2242 ) ;
#10424=EDGE_CURVE ( 'NONE', #5079, #11951, #12754, .T. ) ;
#10425=VERTEX_POINT ( 'NONE', #4995 ) ;
#10437=CARTESIAN_POINT ( 'NONE',  ( 2.449293598294706513E-15, -20.00000000000000000, -8.999999999999998224 ) ) ;
#10446=DIRECTION ( 'NONE',  ( -9.858538378746663627E-23, 5.031452844637890958E-23, -1.000000000000000000 ) ) ;
#10451=CARTESIAN_POINT ( 'NONE',  ( 2.449293598294706513E-15, -20.00000000000000000, 15.00000000000000355 ) ) ;
#10454=EDGE_CURVE ( 'NONE', #10906, #6800, #1720, .T. ) ;
#10482=FACE_OUTER_BOUND ( 'NONE', #3755, .T. ) ;
#10494=ADVANCED_FACE ( 'NONE', ( #2840 ), #4925, .F. ) ;
#10497=ADVANCED_FACE ( 'NONE', ( #10092 ), #11059, .T. ) ;
#10507=PLANE ( 'NONE',  #4845 ) ;
#10508=VECTOR ( 'NONE', #8588, 1000.000000000000000 ) ;
#10531=EDGE_CURVE ( 'NONE', #9171, #6905, #12086, .T. ) ;
#10534=FACE_OUTER_BOUND ( 'NONE', #7360, .T. ) ;
#10545=LINE ( 'NONE', #5307, #666 ) ;
#10550=CARTESIAN_POINT ( 'NONE',  ( 2.449293598294706513E-15, -20.00000000000000000, -9.999999999999994671 ) ) ;
#10556=ORIENTED_EDGE ( 'NONE', *, *, #1611, .T. ) ;
#10560=DIRECTION ( 'NONE',  ( -0.6520673188974834833, 0.7581610723493046322, 1.805535875966852419E-17 ) ) ;
#10561=CARTESIAN_POINT ( 'NONE',  ( 2.449293598294706513E-15, -20.00000000000000000, -20.00000000000000000 ) ) ;
#10567=STYLED_ITEM('',(#13719),#5785);
#10571=ORIENTED_EDGE ( 'NONE', *, *, #4620, .T. ) ;
#10587=EDGE_LOOP ( 'NONE', ( #1081, #8728, #12972, #4321 ) ) ;
#10591=ORIENTED_EDGE ( 'NONE', *, *, #3246, .T. ) ;
#10593=CARTESIAN_POINT ( 'NONE',  ( 0.8816464618332836567, -24.71833652004169934, 9.999999999999998224 ) ) ;
#10603=CARTESIAN_POINT ( 'NONE',  ( -4.999999999999998224, -20.00000000000000000, 9.000000000000000000 ) ) ;
#10608=CARTESIAN_POINT ( 'NONE',  ( -22.14999999999999858, -19.99999999999999289, -23.00000000000000000 ) ) ;
#10611=ORIENTED_EDGE ( 'NONE', *, *, #10531, .F. ) ;
#10615=CARTESIAN_POINT ( 'NONE',  ( 20.00000000000000000, -25.00000000000000711, -23.00000000000000000 ) ) ;
#10621=CARTESIAN_POINT ( 'NONE',  ( 2.449293598294706513E-15, -20.00000000000000000, 15.00000000000000355 ) ) ;
#10626=CIRCLE ( 'NONE', #7335, 5.000000000000007994 ) ;
#10658=EDGE_CURVE ( 'NONE', #3147, #4780, #13114, .T. ) ;
#10663=EDGE_CURVE ( 'NONE', #10425, #1787, #7696, .T. ) ;
#10673=DIRECTION ( 'NONE',  ( -0.000000000000000000, -0.000000000000000000, -1.000000000000000000 ) ) ;
#10699=VECTOR ( 'NONE', #424, 1000.000000000000114 ) ;
#10706=CARTESIAN_POINT ( 'NONE',  ( -14.14213562373094746, -25.00000000000000000, -23.00000000000000000 ) ) ;
#10724=DIRECTION ( 'NONE',  ( -0.9768494444668812671, -0.2139279384389642935, 0.000000000000000000 ) ) ;
#10737=EDGE_CURVE ( 'NONE', #504, #12170, #11667, .T. ) ;
#10746=DIRECTION ( 'NONE',  ( -9.710251638871371392E-17, -5.969973981896233748E-17, -1.000000000000000000 ) ) ;
#10751=DIRECTION ( 'NONE',  ( -0.7779254092217071648, -0.6283566325640553840, 1.130512422757410748E-16 ) ) ;
#10762=FACE_BOUND ( 'NONE', #12024, .T. ) ;
#10770=ADVANCED_FACE ( 'NONE', ( #1987 ), #13312, .F. ) ;
#10772=DIRECTION ( 'NONE',  ( 9.858538378746663627E-23, -5.031452844637890958E-23, 1.000000000000000000 ) ) ;
#10776=DIRECTION ( 'NONE',  ( -0.000000000000000000, -0.000000000000000000, -1.000000000000000000 ) ) ;
#10781=VECTOR ( 'NONE', #10941, 1000.000000000000000 ) ;
#10782=ORIENTED_EDGE ( 'NONE', *, *, #1693, .F. ) ;
#10817=VERTEX_POINT ( 'NONE', #12567 ) ;
#10821=( GEOMETRIC_REPRESENTATION_CONTEXT ( 3 ) GLOBAL_UNCERTAINTY_ASSIGNED_CONTEXT ( ( #13092 ) ) GLOBAL_UNIT_ASSIGNED_CONTEXT ( ( #10859, #8793, #5551 ) ) REPRESENTATION_CONTEXT ( 'NONE', 'WORKASPACE' ) );
#10822=AXIS2_PLACEMENT_3D ( 'NONE', #542, #7964, #6997 ) ;
#10833=LINE ( 'NONE', #7405, #3792 ) ;
#10837=VERTEX_POINT ( 'NONE', #8626 ) ;
#10842=CARTESIAN_POINT ( 'NONE',  ( 20.00000000000000000, -20.00000000000000000, -23.00000000000000000 ) ) ;
#10844=DIRECTION ( 'NONE',  ( -0.9768494444668812671, -0.2139279384389642935, 0.000000000000000000 ) ) ;
#10859=( LENGTH_UNIT ( ) NAMED_UNIT ( * ) SI_UNIT ( .MILLI., .METRE. ) );
#10870=CARTESIAN_POINT ( 'NONE',  ( 20.00000000000000000, -14.99999999999999289, -20.00000000000000000 ) ) ;
#10880=FACE_OUTER_BOUND ( 'NONE', #5751, .T. ) ;
#10881=CYLINDRICAL_SURFACE ( 'NONE', #2850, 4.800000000000000711 ) ;
#10885=ORIENTED_EDGE ( 'NONE', *, *, #7173, .T. ) ;
#10897=DIRECTION ( 'NONE',  ( 0.7969485188038759604, 0.6040472319084893016, -1.134471691914156900E-16 ) ) ;
#10901=VECTOR ( 'NONE', #10252, 1000.000000000000000 ) ;
#10903=ORIENTED_EDGE ( 'NONE', *, *, #8399, .F. ) ;
#10906=VERTEX_POINT ( 'NONE', #7394 ) ;
#10910=ADVANCED_FACE ( 'NONE', ( #12698 ), #6889, .T. ) ;
#10912=DIRECTION ( 'NONE',  ( 9.710251638871371392E-17, 5.969973981896233748E-17, 1.000000000000000000 ) ) ;
#10915=CIRCLE ( 'NONE', #1408, 15.00000000000000000 ) ;
#10941=DIRECTION ( 'NONE',  ( -0.000000000000000000, -0.000000000000000000, 1.000000000000000000 ) ) ;
#10955=VERTEX_POINT ( 'NONE', #3702 ) ;
#10973=DIRECTION ( 'NONE',  ( -1.000000000000000000, 0.000000000000000000, 0.000000000000000000 ) ) ;
#10974=ORIENTED_EDGE ( 'NONE', *, *, #2293, .F. ) ;
#10990=DIRECTION ( 'NONE',  ( 0.000000000000000000, 0.000000000000000000, 1.000000000000000000 ) ) ;
#11007=CIRCLE ( 'NONE', #6825, 5.000000000000000888 ) ;
#11008=DIRECTION ( 'NONE',  ( -0.9768494444668812671, -0.2139279384389642935, 0.000000000000000000 ) ) ;
#11015=DIRECTION ( 'NONE',  ( -1.000000000000000000, 0.000000000000000000, 0.000000000000000000 ) ) ;
#11016=CARTESIAN_POINT ( 'NONE',  ( 0.000000000000000000, 0.000000000000000000, 8.999999999999998224 ) ) ;
#11026=LINE ( 'NONE', #4750, #1555 ) ;
#11036=SHAPE_REPRESENTATION ( 'motor', ( #430 ), #10821 ) ;
#11059=CYLINDRICAL_SURFACE ( 'NONE', #2603, 15.00000000000000000 ) ;
#11068=AXIS2_PLACEMENT_3D ( 'NONE', #110, #3291, #10751 ) ;
#11074=EDGE_LOOP ( 'NONE', ( #6214, #5419, #11618, #11861 ) ) ;
#11095=ORIENTED_EDGE ( 'NONE', *, *, #6753, .F. ) ;
#11099=DIRECTION ( 'NONE',  ( -1.000000000000000000, 0.000000000000000000, 0.000000000000000000 ) ) ;
#11101=CARTESIAN_POINT ( 'NONE',  ( 25.00000000000000711, -20.00000000000000000, -23.00000000000000000 ) ) ;
#11124=VECTOR ( 'NONE', #2870, 1000.000000000000000 ) ;
#11143=CIRCLE ( 'NONE', #8718, 15.00000000000000000 ) ;
#11147=EDGE_CURVE ( 'NONE', #5892, #9150, #11007, .T. ) ;
#11150=FACE_OUTER_BOUND ( 'NONE', #11632, .T. ) ;
#11180=EDGE_LOOP ( 'NONE', ( #4714, #2908, #118, #2755, #7486, #3890, #4286, #10885 ) ) ;
#11198=DIRECTION ( 'NONE',  ( 0.000000000000000000, 0.000000000000000000, -1.000000000000000000 ) ) ;
#11202=DIRECTION ( 'NONE',  ( 0.000000000000000000, 0.000000000000000000, -1.000000000000000000 ) ) ;
#11216=LINE ( 'NONE', #13350, #10901 ) ;
#11231=ORIENTED_EDGE ( 'NONE', *, *, #5188, .T. ) ;
#11237=CARTESIAN_POINT ( 'NONE',  ( 2.482347295856823136E-15, -20.00000000000000000, -8.999999999999996447 ) ) ;
#11255=VERTEX_POINT ( 'NONE', #6414 ) ;
#11257=CARTESIAN_POINT ( 'NONE',  ( 22.14999999999999858, -20.00000000000000000, -23.00000000000000000 ) ) ;
#11265=DIRECTION ( 'NONE',  ( -9.710251638871371392E-17, -5.969973981896233748E-17, -1.000000000000000000 ) ) ;
#11281=DIRECTION ( 'NONE',  ( 0.000000000000000000, 0.000000000000000000, 1.000000000000000000 ) ) ;
#11322=EDGE_CURVE ( 'NONE', #10955, #11356, #12562, .T. ) ;
#11323=CARTESIAN_POINT ( 'NONE',  ( 20.00000000000000000, -25.00000000000000711, -20.00000000000000000 ) ) ;
#11333=DIRECTION ( 'NONE',  ( -9.858538378746663627E-23, 5.031452844637890958E-23, -1.000000000000000000 ) ) ;
#11341=ORIENTED_EDGE ( 'NONE', *, *, #4336, .F. ) ;
#11346=FACE_OUTER_BOUND ( 'NONE', #5906, .T. ) ;
#11356=VERTEX_POINT ( 'NONE', #2233 ) ;
#11375=DIRECTION ( 'NONE',  ( -0.000000000000000000, -0.000000000000000000, -1.000000000000000000 ) ) ;
#11378=CARTESIAN_POINT ( 'NONE',  ( 14.14213562373095101, -25.00000000000000711, -20.00000000000000000 ) ) ;
#11433=EDGE_CURVE ( 'NONE', #4979, #8761, #8029, .T. ) ;
#11435=CARTESIAN_POINT ( 'NONE',  ( -14.99999999999999822, -19.99999999999999645, -50.00000000000000000 ) ) ;
#11440=DIRECTION ( 'NONE',  ( -9.858538378746663627E-23, 5.031452844637890958E-23, -1.000000000000000000 ) ) ;
#11460=AXIS2_PLACEMENT_3D ( 'NONE', #7054, #11265, #3431 ) ;
#11479=CIRCLE ( 'NONE', #13006, 4.800000000000000711 ) ;
#11517=DIRECTION ( 'NONE',  ( 9.858538378746663627E-23, -5.031452844637890958E-23, 1.000000000000000000 ) ) ;
#11540=EDGE_CURVE ( 'NONE', #11760, #12920, #743, .T. ) ;
#11542=EDGE_CURVE ( 'NONE', #13537, #2771, #8809, .T. ) ;
#11544=DIRECTION ( 'NONE',  ( -1.000000000000000000, 0.000000000000000000, -0.000000000000000000 ) ) ;
#11545=AXIS2_PLACEMENT_3D ( 'NONE', #8313, #5338, #9414 ) ;
#11555=VERTEX_POINT ( 'NONE', #5965 ) ;
#11557=DIRECTION ( 'NONE',  ( 0.000000000000000000, 0.000000000000000000, -1.000000000000000000 ) ) ;
#11560=LINE ( 'NONE', #2070, #470 ) ;
#11568=ORIENTED_EDGE ( 'NONE', *, *, #10663, .T. ) ;
#11584=CARTESIAN_POINT ( 'NONE',  ( -1.000000000000000000, -14.00000000000000000, 8.999999999999998224 ) ) ;
#11593=LINE ( 'NONE', #7575, #11727 ) ;
#11609=FACE_OUTER_BOUND ( 'NONE', #3331, .T. ) ;
#11618=ORIENTED_EDGE ( 'NONE', *, *, #5192, .T. ) ;
#11632=EDGE_LOOP ( 'NONE', ( #12038, #10591 ) ) ;
#11640=CARTESIAN_POINT ( 'NONE',  ( -20.00000000000000000, -19.99999999999999289, -23.00000000000000000 ) ) ;
#11667=CIRCLE ( 'NONE', #8146, 2.149999999999999023 ) ;
#11677=CARTESIAN_POINT ( 'NONE',  ( -0.9999999999999995559, -15.10102051443364246, -8.999999999999998224 ) ) ;
#11702=LINE ( 'NONE', #2225, #11740 ) ;
#11715=CARTESIAN_POINT ( 'NONE',  ( 15.00000000000000178, -20.00000000000000000, -50.00000000000000000 ) ) ;
#11727=VECTOR ( 'NONE', #11783, 1000.000000000000000 ) ;
#11730=ORIENTED_EDGE ( 'NONE', *, *, #281, .F. ) ;
#11732=LINE ( 'NONE', #6500, #1880 ) ;
#11740=VECTOR ( 'NONE', #10673, 1000.000000000000000 ) ;
#11759=ADVANCED_FACE ( 'NONE', ( #7347 ), #10507, .T. ) ;
#11760=VERTEX_POINT ( 'NONE', #1020 ) ;
#11773=FACE_OUTER_BOUND ( 'NONE', #11074, .T. ) ;
#11783=DIRECTION ( 'NONE',  ( -9.858538378746663627E-23, 5.031452844637890958E-23, -1.000000000000000000 ) ) ;
#11789=DIRECTION ( 'NONE',  ( -9.858538378746663627E-23, 5.031452844637890958E-23, -1.000000000000000000 ) ) ;
#11808=DIRECTION ( 'NONE',  ( -0.6520673188974834833, 0.7581610723493047432, 1.805535875966851803E-17 ) ) ;
#11823=VERTEX_POINT ( 'NONE', #2134 ) ;
#11843=PLANE ( 'NONE',  #9040 ) ;
#11845=CARTESIAN_POINT ( 'NONE',  ( -14.99999999999999822, -19.99999999999999645, -50.00000000000000000 ) ) ;
#11861=ORIENTED_EDGE ( 'NONE', *, *, #6753, .T. ) ;
#11863=ORIENTED_EDGE ( 'NONE', *, *, #7525, .T. ) ;
#11867=DIRECTION ( 'NONE',  ( -0.000000000000000000, -0.000000000000000000, -1.000000000000000000 ) ) ;
#11922=DIRECTION ( 'NONE',  ( -0.000000000000000000, -0.000000000000000000, 1.000000000000000000 ) ) ;
#11925=PLANE ( 'NONE',  #100 ) ;
#11926=EDGE_CURVE ( 'NONE', #347, #12678, #333, .T. ) ;
#11944=VECTOR ( 'NONE', #6482, 1000.000000000000000 ) ;
#11945=EDGE_CURVE ( 'NONE', #4523, #4643, #13568, .T. ) ;
#11949=ORIENTED_EDGE ( 'NONE', *, *, #5425, .T. ) ;
#11951=VERTEX_POINT ( 'NONE', #11677 ) ;
#11981=CIRCLE ( 'NONE', #4478, 5.000000000000000888 ) ;
#11985=ORIENTED_EDGE ( 'NONE', *, *, #9719, .F. ) ;
#11992=LINE ( 'NONE', #1324, #3556 ) ;
#11997=FACE_OUTER_BOUND ( 'NONE', #6121, .T. ) ;
#11998=FACE_OUTER_BOUND ( 'NONE', #9624, .T. ) ;
#12001=DIRECTION ( 'NONE',  ( 1.734723475976806848E-16, 1.000000000000000000, 0.000000000000000000 ) ) ;
#12003=ORIENTED_EDGE ( 'NONE', *, *, #3479, .F. ) ;
#12023=CARTESIAN_POINT ( 'NONE',  ( 20.00000000000000000, -20.00000000000000000, -23.00000000000000000 ) ) ;
#12024=EDGE_LOOP ( 'NONE', ( #2624, #405 ) ) ;
#12034=EDGE_CURVE ( 'NONE', #11555, #13173, #4906, .T. ) ;
#12038=ORIENTED_EDGE ( 'NONE', *, *, #3170, .T. ) ;
#12040=ORIENTED_EDGE ( 'NONE', *, *, #12827, .T. ) ;
#12050=FACE_OUTER_BOUND ( 'NONE', #4119, .T. ) ;
#12056=ORIENTED_EDGE ( 'NONE', *, *, #3817, .T. ) ;
#12086=LINE ( 'NONE', #5876, #10103 ) ;
#12095=DIRECTION ( 'NONE',  ( -0.000000000000000000, -0.000000000000000000, 1.000000000000000000 ) ) ;
#12117=( GEOMETRIC_REPRESENTATION_CONTEXT ( 3 ) GLOBAL_UNCERTAINTY_ASSIGNED_CONTEXT ( ( #5153 ) ) GLOBAL_UNIT_ASSIGNED_CONTEXT ( ( #4129, #3913, #9313 ) ) REPRESENTATION_CONTEXT ( 'NONE', 'WORKASPACE' ) );
#12119=DIRECTION ( 'NONE',  ( 1.000000000000000000, -1.734723475976807341E-16, -0.000000000000000000 ) ) ;
#12126=AXIS2_PLACEMENT_3D ( 'NONE', #294, #4449, #12871 ) ;
#12135=ORIENTED_EDGE ( 'NONE', *, *, #9145, .F. ) ;
#12170=VERTEX_POINT ( 'NONE', #1704 ) ;
#12172=VERTEX_POINT ( 'NONE', #524 ) ;
#12193=DIRECTION ( 'NONE',  ( 1.000000000000000000, 0.000000000000000000, -0.000000000000000000 ) ) ;
#12198=DIRECTION ( 'NONE',  ( -1.000000000000000000, 0.000000000000000000, 0.000000000000000000 ) ) ;
#12208=CARTESIAN_POINT ( 'NONE',  ( 5.000000000000003553, -20.00000000000000000, -8.999999999999998224 ) ) ;
#12223=VERTEX_POINT ( 'NONE', #11323 ) ;
#12234=VERTEX_POINT ( 'NONE', #869 ) ;
#12235=ORIENTED_EDGE ( 'NONE', *, *, #2109, .T. ) ;
#12236=EDGE_CURVE ( 'NONE', #407, #13146, #11143, .T. ) ;
#12237=ORIENTED_EDGE ( 'NONE', *, *, #12761, .F. ) ;
#12251=DIRECTION ( 'NONE',  ( -0.7779254092217071648, -0.6283566325640553840, 0.000000000000000000 ) ) ;
#12254=ORIENTED_EDGE ( 'NONE', *, *, #13406, .F. ) ;
#12258=CARTESIAN_POINT ( 'NONE',  ( 20.00000000000000000, -25.00000000000000711, -20.00000000000000000 ) ) ;
#12266=DIRECTION ( 'NONE',  ( 0.000000000000000000, 0.000000000000000000, -1.000000000000000000 ) ) ;
#12269=CARTESIAN_POINT ( 'NONE',  ( 20.00000000000000000, -20.00000000000000000, -20.00000000000000000 ) ) ;
#12283=CARTESIAN_POINT ( 'NONE',  ( 4.688877333453707941, -18.97314589549297281, 9.999999999999998224 ) ) ;
#12292=EDGE_CURVE ( 'NONE', #2771, #13537, #13122, .T. ) ;
#12318=ORIENTED_EDGE ( 'NONE', *, *, #13444, .T. ) ;
#12326=AXIS2_PLACEMENT_3D ( 'NONE', #12023, #6770, #10973 ) ;
#12348=EDGE_CURVE ( 'NONE', #11555, #12722, #10915, .T. ) ;
#12351=EDGE_CURVE ( 'NONE', #13245, #2677, #4975, .T. ) ;
#12363=FACE_OUTER_BOUND ( 'NONE', #10587, .T. ) ;
#12374=ORIENTED_EDGE ( 'NONE', *, *, #7184, .T. ) ;
#12376=DIRECTION ( 'NONE',  ( 1.734723475976806848E-16, 1.000000000000000000, 0.000000000000000000 ) ) ;
#12394=CARTESIAN_POINT ( 'NONE',  ( 2.385244779468109755E-15, -20.00000000000000000, -9.999999999999994671 ) ) ;
#12403=DIRECTION ( 'NONE',  ( -0.9768494444668812671, -0.2139279384389642935, 0.000000000000000000 ) ) ;
#12414=CARTESIAN_POINT ( 'NONE',  ( 2.482347295856823136E-15, -20.00000000000000000, -8.999999999999996447 ) ) ;
#12421=VECTOR ( 'NONE', #13200, 1000.000000000000000 ) ;
#12428=AXIS2_PLACEMENT_3D ( 'NONE', #7055, #11333, #735 ) ;
#12429=CARTESIAN_POINT ( 'NONE',  ( -0.9999999999999976685, -20.00000000000000000, 8.999999999999998224 ) ) ;
#12444=CARTESIAN_POINT ( 'NONE',  ( 2.899426713160750069, -23.82535289025860337, -9.999999999999994671 ) ) ;
#12469=VECTOR ( 'NONE', #2543, 1000.000000000000000 ) ;
#12471=DIRECTION ( 'NONE',  ( 0.000000000000000000, 0.000000000000000000, -1.000000000000000000 ) ) ;
#12475=CARTESIAN_POINT ( 'NONE',  ( 1.267864665261691752E-11, -20.00000000000000000, 9.999999999999998224 ) ) ;
#12479=VERTEX_POINT ( 'NONE', #9732 ) ;
#12496=ORIENTED_EDGE ( 'NONE', *, *, #9897, .T. ) ;
#12498=LINE ( 'NONE', #13453, #5630 ) ;
#12500=CIRCLE ( 'NONE', #12711, 2.149999999999999023 ) ;
#12511=VERTEX_POINT ( 'NONE', #3239 ) ;
#12525=EDGE_CURVE ( 'NONE', #651, #13554, #11732, .T. ) ;
#12532=CARTESIAN_POINT ( 'NONE',  ( -4.999999999999998224, -20.00000000000000000, -9.999999999999994671 ) ) ;
#12557=LINE ( 'NONE', #10413, #2420 ) ;
#12562=CIRCLE ( 'NONE', #13207, 15.00000000000000000 ) ;
#12566=ORIENTED_EDGE ( 'NONE', *, *, #9580, .F. ) ;
#12567=CARTESIAN_POINT ( 'NONE',  ( 15.00000000000000178, -20.00000000000000000, -50.00000000000000000 ) ) ;
#12578=ORIENTED_EDGE ( 'NONE', *, *, #13172, .F. ) ;
#12584=FACE_OUTER_BOUND ( 'NONE', #13112, .T. ) ;
#12603=EDGE_CURVE ( 'NONE', #690, #11255, #2284, .T. ) ;
#12616=DIRECTION ( 'NONE',  ( 0.000000000000000000, 0.000000000000000000, -1.000000000000000000 ) ) ;
#12618=PRODUCT_DEFINITION_SHAPE ( 'NONE', 'NONE',  #9454 ) ;
#12635=CARTESIAN_POINT ( 'NONE',  ( 3.129923130707922496, -23.63917314727666152, -8.999999999999996447 ) ) ;
#12645=ORIENTED_EDGE ( 'NONE', *, *, #12292, .F. ) ;
#12648=DIRECTION ( 'NONE',  ( -1.000000000000000000, 0.000000000000000000, -0.000000000000000000 ) ) ;
#12674=CIRCLE ( 'NONE', #1628, 15.00000000000000000 ) ;
#12677=AXIS2_PLACEMENT_3D ( 'NONE', #2098, #11517, #12403 ) ;
#12678=VERTEX_POINT ( 'NONE', #12208 ) ;
#12689=VECTOR ( 'NONE', #3781, 1000.000000000000000 ) ;
#12698=FACE_OUTER_BOUND ( 'NONE', #4991, .T. ) ;
#12711=AXIS2_PLACEMENT_3D ( 'NONE', #3834, #5852, #11015 ) ;
#12713=EDGE_CURVE ( 'NONE', #12234, #6107, #9614, .T. ) ;
#12715=CARTESIAN_POINT ( 'NONE',  ( 3.129923130707922496, -23.63917314727666152, -8.999999999999996447 ) ) ;
#12719=DIRECTION ( 'NONE',  ( -0.6520673188974834833, 0.7581610723493047432, 1.805535875966851803E-17 ) ) ;
#12722=VERTEX_POINT ( 'NONE', #5102 ) ;
#12742=DIRECTION ( 'NONE',  ( -0.7779254092217071648, -0.6283566325640553840, 0.000000000000000000 ) ) ;
#12744=DIRECTION ( 'NONE',  ( 1.000000000000000000, 0.000000000000000000, 0.000000000000000000 ) ) ;
#12747=LINE ( 'NONE', #1203, #9756 ) ;
#12751=ADVANCED_BREP_SHAPE_REPRESENTATION ( '', ( #5785, #430 ), #10821 ) ;
#12754=CIRCLE ( 'NONE', #5710, 5.000000000000000888 ) ;
#12761=EDGE_CURVE ( 'NONE', #5149, #5888, #8272, .T. ) ;
#12776=AXIS2_PLACEMENT_3D ( 'NONE', #13153, #9230, #4739 ) ;
#12783=LINE ( 'NONE', #3462, #12850 ) ;
#12791=FACE_OUTER_BOUND ( 'NONE', #8587, .T. ) ;
#12819=CARTESIAN_POINT ( 'NONE',  ( 0.8816464618332836567, -24.71833652004169934, 9.000000000000000000 ) ) ;
#12825=ORIENTED_EDGE ( 'NONE', *, *, #6654, .T. ) ;
#12827=EDGE_CURVE ( 'NONE', #3147, #9171, #7244, .T. ) ;
#12832=AXIS2_PLACEMENT_3D ( 'NONE', #1885, #13351, #12193 ) ;
#12835=AXIS2_PLACEMENT_3D ( 'NONE', #2569, #2500, #5558 ) ;
#12840=VERTEX_POINT ( 'NONE', #784 ) ;
#12850=VECTOR ( 'NONE', #12719, 999.9999999999998863 ) ;
#12853=ORIENTED_EDGE ( 'NONE', *, *, #10424, .T. ) ;
#12858=CARTESIAN_POINT ( 'NONE',  ( 2.449293598294706513E-15, -20.00000000000000000, 15.00000000000000355 ) ) ;
#12871=DIRECTION ( 'NONE',  ( -1.000000000000000000, 0.000000000000000000, 0.000000000000000000 ) ) ;
#12879=CARTESIAN_POINT ( 'NONE',  ( 20.00000000000000000, -20.00000000000000000, -23.00000000000000000 ) ) ;
#12882=CYLINDRICAL_SURFACE ( 'NONE', #3353, 5.000000000000000888 ) ;
#12895=FACE_OUTER_BOUND ( 'NONE', #4502, .T. ) ;
#12901=PLANE ( 'NONE',  #13449 ) ;
#12920=VERTEX_POINT ( 'NONE', #4191 ) ;
#12939=ORIENTED_EDGE ( 'NONE', *, *, #2542, .T. ) ;
#12946=FACE_OUTER_BOUND ( 'NONE', #11180, .T. ) ;
#12958=CYLINDRICAL_SURFACE ( 'NONE', #5557, 5.000000000000000888 ) ;
#12966=DIRECTION ( 'NONE',  ( -9.858538378746663627E-23, 5.031452844637890958E-23, -1.000000000000000000 ) ) ;
#12971=VERTEX_POINT ( 'NONE', #4454 ) ;
#12972=ORIENTED_EDGE ( 'NONE', *, *, #12603, .F. ) ;
#12992=ORIENTED_EDGE ( 'NONE', *, *, #2013, .F. ) ;
#13006=AXIS2_PLACEMENT_3D ( 'NONE', #5475, #5744, #10844 ) ;
#13008=EDGE_CURVE ( 'NONE', #11823, #8572, #5243, .T. ) ;
#13011=ADVANCED_FACE ( 'NONE', ( #4385 ), #8610, .F. ) ;
#13029=AXIS2_PLACEMENT_3D ( 'NONE', #7899, #10172, #5065 ) ;
#13031=DIRECTION ( 'NONE',  ( -0.000000000000000000, -0.000000000000000000, -1.000000000000000000 ) ) ;
#13044=ORIENTED_EDGE ( 'NONE', *, *, #260, .F. ) ;
#13053=CARTESIAN_POINT ( 'NONE',  ( -14.14213562373094746, -25.00000000000000000, -50.00000000000000000 ) ) ;
#13071=AXIS2_PLACEMENT_3D ( 'NONE', #610, #13273, #12251 ) ;
#13074=LINE ( 'NONE', #6932, #12421 ) ;
#13090=LINE ( 'NONE', #13361, #11124 ) ;
#13092=UNCERTAINTY_MEASURE_WITH_UNIT (LENGTH_MEASURE( 1.000000000000000082E-05 ), #10859, 'distance_accuracy_value', 'NONE');
#13112=EDGE_LOOP ( 'NONE', ( #10611, #11949, #31, #823, #8257, #4938, #7110, #2659, #346, #12853, #3026, #10571 ) ) ;
#13114=LINE ( 'NONE', #3588, #3054 ) ;
#13119=DIRECTION ( 'NONE',  ( 0.1836763462126260738, -0.9829867750086873635, -1.521953536530129477E-22 ) ) ;
#13121=LINE ( 'NONE', #3458, #9045 ) ;
#13122=CIRCLE ( 'NONE', #1199, 2.149999999999999023 ) ;
#13127=ORIENTED_EDGE ( 'NONE', *, *, #4163, .T. ) ;
#13130=ORIENTED_EDGE ( 'NONE', *, *, #12827, .F. ) ;
#13134=CARTESIAN_POINT ( 'NONE',  ( 20.00000000000000000, -14.99999999999999289, -23.00000000000000000 ) ) ;
#13146=VERTEX_POINT ( 'NONE', #5775 ) ;
#13152=CARTESIAN_POINT ( 'NONE',  ( 1.000000000000000000, -14.00000000000000000, 8.999999999999998224 ) ) ;
#13153=CARTESIAN_POINT ( 'NONE',  ( 2.449293598294706513E-15, -20.00000000000000000, -50.00000000000000000 ) ) ;
#13161=DIRECTION ( 'NONE',  ( 0.000000000000000000, 0.000000000000000000, -1.000000000000000000 ) ) ;
#13172=EDGE_CURVE ( 'NONE', #8572, #12920, #6940, .T. ) ;
#13173=VERTEX_POINT ( 'NONE', #3688 ) ;
#13179=EDGE_CURVE ( 'NONE', #4979, #10817, #12674, .T. ) ;
#13200=DIRECTION ( 'NONE',  ( -0.000000000000000000, -0.000000000000000000, 1.000000000000000000 ) ) ;
#13206=EDGE_CURVE ( 'NONE', #12920, #10164, #8495, .T. ) ;
#13207=AXIS2_PLACEMENT_3D ( 'NONE', #3083, #12616, #8477 ) ;
#13208=CARTESIAN_POINT ( 'NONE',  ( 2.449293598294706513E-15, -20.00000000000000000, -50.00000000000000000 ) ) ;
#13221=DIRECTION ( 'NONE',  ( -0.000000000000000000, -0.000000000000000000, -1.000000000000000000 ) ) ;
#13223=AXIS2_PLACEMENT_3D ( 'NONE', #2574, #2853, #10106 ) ;
#13225=ORIENTED_EDGE ( 'NONE', *, *, #360, .T. ) ;
#13229=AXIS2_PLACEMENT_3D ( 'NONE', #385, #12966, #9668 ) ;
#13235=CARTESIAN_POINT ( 'NONE',  ( -1.000000000000000000, -14.00000000000000000, -9.000000000000001776 ) ) ;
#13245=VERTEX_POINT ( 'NONE', #9907 ) ;
#13263=DIRECTION ( 'NONE',  ( 1.000000000000000000, 0.000000000000000000, 0.000000000000000000 ) ) ;
#13270=AXIS2_PLACEMENT_3D ( 'NONE', #6942, #3893, #3757 ) ;
#13272=AXIS2_PLACEMENT_3D ( 'NONE', #9769, #4515, #6797 ) ;
#13273=DIRECTION ( 'NONE',  ( -9.710251638871371392E-17, -5.969973981896233748E-17, -1.000000000000000000 ) ) ;
#13275=EDGE_CURVE ( 'NONE', #12511, #12971, #1855, .T. ) ;
#13301=CARTESIAN_POINT ( 'NONE',  ( 1.000000000000000000, -14.00000000000000000, -9.000000000000001776 ) ) ;
#13311=EDGE_LOOP ( 'NONE', ( #1681, #7169, #845, #7314 ) ) ;
#13312=PLANE ( 'NONE',  #9462 ) ;
#13315=CARTESIAN_POINT ( 'NONE',  ( 0.8816464618332836567, -24.71833652004169934, 9.000000000000000000 ) ) ;
#13330=DIRECTION ( 'NONE',  ( -9.710251638871371392E-17, -5.969973981896233748E-17, -1.000000000000000000 ) ) ;
#13346=EDGE_CURVE ( 'NONE', #8761, #13173, #9807, .T. ) ;
#13350=CARTESIAN_POINT ( 'NONE',  ( 14.14213562373094923, -14.99999999999999112, -50.00000000000000000 ) ) ;
#13351=DIRECTION ( 'NONE',  ( 0.000000000000000000, 0.000000000000000000, 1.000000000000000000 ) ) ;
#13352=EDGE_CURVE ( 'NONE', #5185, #5079, #10392, .T. ) ;
#13357=LINE ( 'NONE', #13152, #5134 ) ;
#13361=CARTESIAN_POINT ( 'NONE',  ( -19.99999999999999289, -14.99999999999998579, -23.00000000000000000 ) ) ;
#13366=VECTOR ( 'NONE', #6412, 1000.000000000000000 ) ;
#13380=ORIENTED_EDGE ( 'NONE', *, *, #995, .F. ) ;
#13383=DIRECTION ( 'NONE',  ( 0.000000000000000000, 0.000000000000000000, -1.000000000000000000 ) ) ;
#13398=DIRECTION ( 'NONE',  ( -1.000000000000000000, 0.000000000000000000, 0.000000000000000000 ) ) ;
#13406=EDGE_CURVE ( 'NONE', #3770, #12722, #11216, .T. ) ;
#13418=APPLICATION_CONTEXT ( 'automotive_design' ) ;
#13423=MECHANICAL_DESIGN_GEOMETRIC_PRESENTATION_REPRESENTATION('',(#10567),#12117);
#13426=FACE_OUTER_BOUND ( 'NONE', #406, .T. ) ;
#13429=DIRECTION ( 'NONE',  ( 0.000000000000000000, -0.000000000000000000, 1.000000000000000000 ) ) ;
#13436=FACE_OUTER_BOUND ( 'NONE', #1827, .T. ) ;
#13444=EDGE_CURVE ( 'NONE', #13146, #1489, #8048, .T. ) ;
#13449=AXIS2_PLACEMENT_3D ( 'NONE', #9866, #10897, #1416 ) ;
#13453=CARTESIAN_POINT ( 'NONE',  ( 20.00000000000000000, -14.99999999999999289, -20.00000000000000000 ) ) ;
#13458=COLOUR_RGB ( '',0.8941176470588234615, 0.8941176470588234615, 0.8941176470588234615 ) ;
#13460=CARTESIAN_POINT ( 'NONE',  ( 3.129923130707922496, -23.63917314727666152, -8.999999999999996447 ) ) ;
#13468=DIRECTION ( 'NONE',  ( -1.000000000000000000, 0.000000000000000000, -0.000000000000000000 ) ) ;
#13494=DIRECTION ( 'NONE',  ( -1.000000000000000000, 0.000000000000000000, 0.000000000000000000 ) ) ;
#13497=DIRECTION ( 'NONE',  ( -0.9768494444668812671, -0.2139279384389642935, 0.000000000000000000 ) ) ;
#13499=AXIS2_PLACEMENT_3D ( 'NONE', #8442, #9800, #12648 ) ;
#13500=LINE ( 'NONE', #842, #13366 ) ;
#13525=DIRECTION ( 'NONE',  ( -4.082155997157844188E-16, 1.000000000000000000, 0.000000000000000000 ) ) ;
#13537=VERTEX_POINT ( 'NONE', #5225 ) ;
#13540=DIRECTION ( 'NONE',  ( -1.000000000000000000, 0.000000000000000000, -0.000000000000000000 ) ) ;
#13554=VERTEX_POINT ( 'NONE', #9427 ) ;
#13559=CARTESIAN_POINT ( 'NONE',  ( -1.000000000000000000, -14.00000000000000000, -9.000000000000001776 ) ) ;
#13568=CIRCLE ( 'NONE', #108, 4.800000000000000711 ) ;
#13569=CARTESIAN_POINT ( 'NONE',  ( 17.85000000000000142, -20.00000000000000000, -20.00000000000000000 ) ) ;
#13575=CARTESIAN_POINT ( 'NONE',  ( 5.000000000000003553, -20.00000000000000000, 15.00000000000000355 ) ) ;
#13594=DIRECTION ( 'NONE',  ( -1.000000000000000000, 0.000000000000000000, 0.000000000000000000 ) ) ;
#13603=DIRECTION ( 'NONE',  ( -1.000000000000000000, 0.000000000000000000, 0.000000000000000000 ) ) ;
#13609=ORIENTED_EDGE ( 'NONE', *, *, #7519, .F. ) ;
#13621=ORIENTED_EDGE ( 'NONE', *, *, #910, .T. ) ;
#13636=ORIENTED_EDGE ( 'NONE', *, *, #4219, .F. ) ;
#13643=CARTESIAN_POINT ( 'NONE',  ( 2.482347295856823136E-15, -20.00000000000000000, -8.999999999999996447 ) ) ;
#13713=COLOUR_RGB('Off White',0.89,0.88,0.83);
#13714=FILL_AREA_STYLE_COLOUR('',#13713);
#13715=FILL_AREA_STYLE('',(#13714));
#13716=SURFACE_STYLE_FILL_AREA(#13715);
#13717=SURFACE_SIDE_STYLE('',(#13716));
#13718=SURFACE_STYLE_USAGE(.BOTH.,#13717);
#13719=PRESENTATION_STYLE_ASSIGNMENT((#13718));
ENDSEC;
END-ISO-10303-21;
